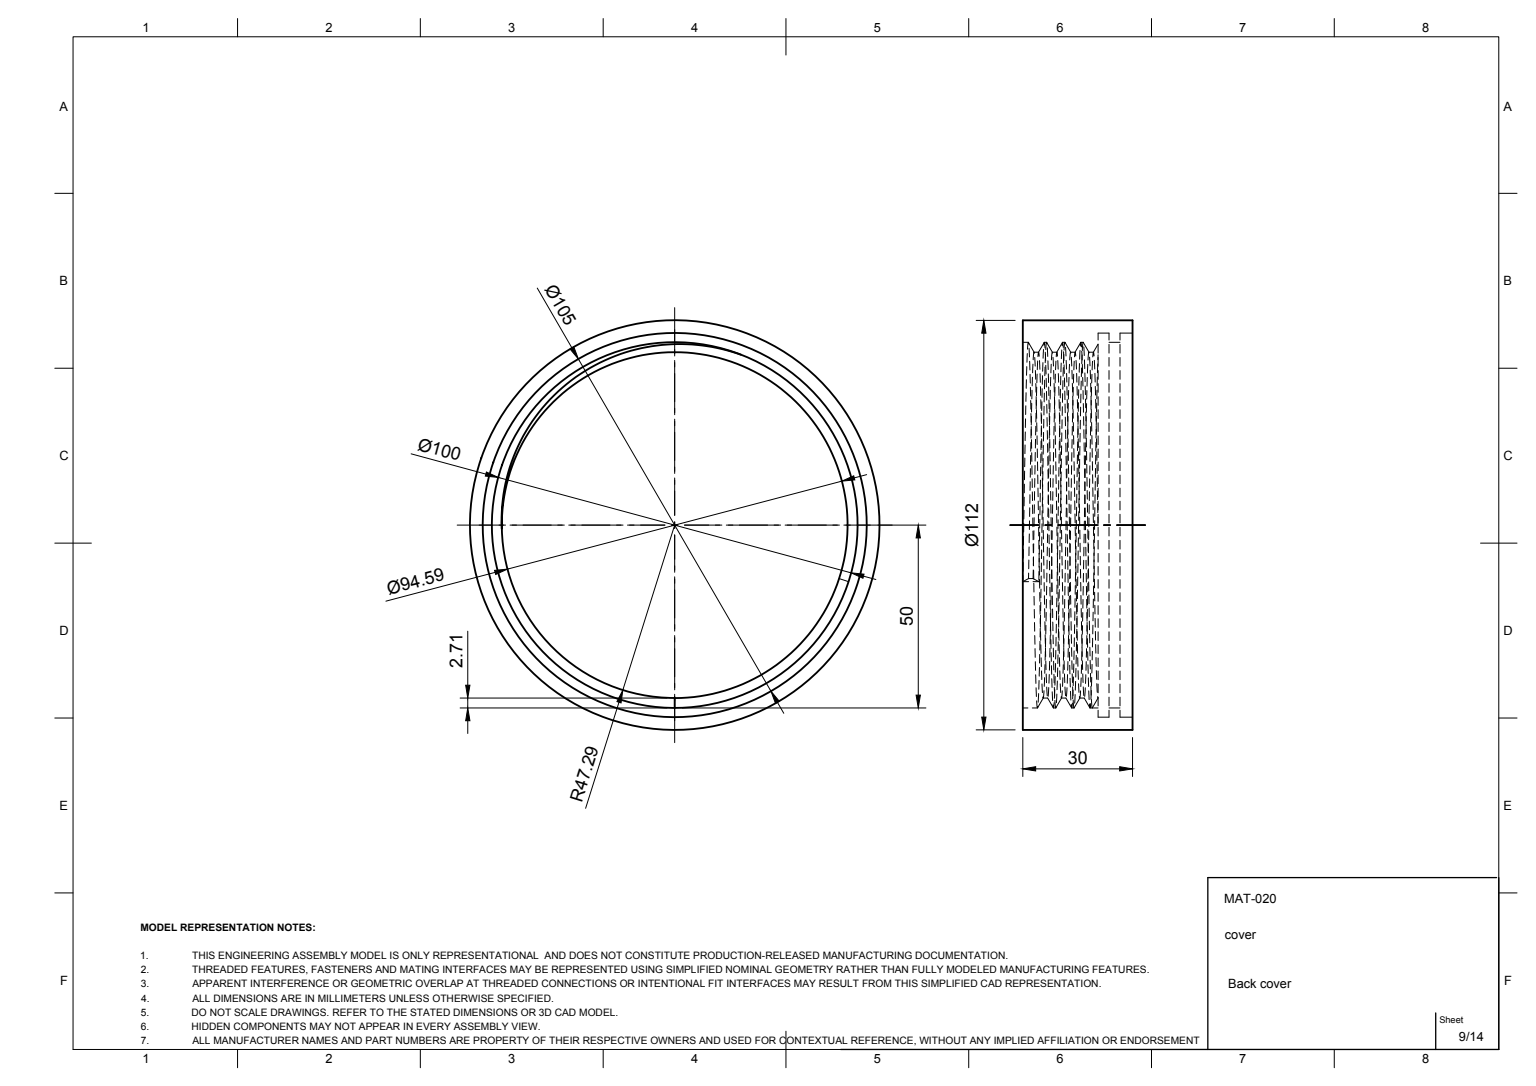
ISO-10303-21;
HEADER;
/* Generated by software containing ST-Developer
 * from STEP Tools, Inc. (www.steptools.com) 
 */

FILE_DESCRIPTION(
/* description */ ('STEP AP214'),
/* implementation_level */ '2;1');

FILE_NAME(
/* name */ 'Cover.step',
/* time_stamp */ '2026-11-14T06:20:50-08:00',
/* author */ (''),
/* organization */ (''),
/* preprocessor_version */ 'ST-DEVELOPER v20.2',
/* originating_system */ 'Autodesk Translation Framework v15.17.0.0',
/* authorisation */ '');

FILE_SCHEMA (('AUTOMOTIVE_DESIGN { 1 0 10303 214 3 1 1 }'));
ENDSEC;

DATA;
#10=MECHANICAL_DESIGN_GEOMETRIC_PRESENTATION_REPRESENTATION('',(#960),#20658);
#127=FACE_BOUND('',#1332,.T.);
#128=FACE_BOUND('',#1334,.T.);
#129=FACE_BOUND('',#1338,.T.);
#130=FACE_BOUND('',#1340,.T.);
#131=FACE_BOUND('',#1342,.T.);
#195=(
BOUNDED_SURFACE()
B_SPLINE_SURFACE(1,2,((#19897,#19898,#19899,#19900,#19901,#19902,#19903,
#19904,#19905,#19906,#19907,#19908,#19909,#19910,#19911,#19912,#19913,#19914,
#19915,#19916,#19917,#19918,#19919,#19920,#19921,#19922,#19923,#19924,#19925,
#19926,#19927,#19928,#19929,#19930,#19931,#19932,#19933,#19934,#19935,#19936,
#19937,#19938,#19939,#19940,#19941,#19942,#19943,#19944,#19945,#19946,#19947,
#19948,#19949,#19950,#19951,#19952,#19953,#19954,#19955,#19956,#19957,#19958,
#19959,#19960,#19961,#19962,#19963,#19964,#19965,#19966,#19967,#19968,#19969,
#19970,#19971,#19972,#19973,#19974,#19975,#19976,#19977,#19978,#19979,#19980,
#19981,#19982,#19983,#19984,#19985,#19986,#19987,#19988,#19989),(#19990,
#19991,#19992,#19993,#19994,#19995,#19996,#19997,#19998,#19999,#20000,#20001,
#20002,#20003,#20004,#20005,#20006,#20007,#20008,#20009,#20010,#20011,#20012,
#20013,#20014,#20015,#20016,#20017,#20018,#20019,#20020,#20021,#20022,#20023,
#20024,#20025,#20026,#20027,#20028,#20029,#20030,#20031,#20032,#20033,#20034,
#20035,#20036,#20037,#20038,#20039,#20040,#20041,#20042,#20043,#20044,#20045,
#20046,#20047,#20048,#20049,#20050,#20051,#20052,#20053,#20054,#20055,#20056,
#20057,#20058,#20059,#20060,#20061,#20062,#20063,#20064,#20065,#20066,#20067,
#20068,#20069,#20070,#20071,#20072,#20073,#20074,#20075,#20076,#20077,#20078,
#20079,#20080,#20081,#20082)),.UNSPECIFIED.,.F.,.F.,.F.)
B_SPLINE_SURFACE_WITH_KNOTS((2,2),(3,2,2,2,2,2,2,2,2,2,2,2,2,2,2,2,2,2,
2,2,2,2,2,2,2,2,2,2,2,2,2,2,2,2,2,2,2,2,2,2,2,2,2,2,2,2,3),(0.,1.),(0.,
0.0208333333333333,0.0416666666666667,0.0625,0.0833333333333333,0.104166666666667,
0.125,0.145833333333333,0.166666666666667,0.1875,0.208333333333333,0.229166666666667,
0.25,0.270833333333333,0.291666666666667,0.3125,0.333333333333333,0.354166666666667,
0.375,0.395833333333333,0.416666666666667,0.4375,0.458333333333333,0.479166666666667,
0.5,0.520833333333333,0.541666666666667,0.5625,0.583333333333333,0.604166666666667,
0.625,0.645833333333333,0.666666666666667,0.6875,0.708333333333333,0.729166666666667,
0.75,0.770833333333333,0.791666666666667,0.8125,0.833333333333333,0.854166666666667,
0.875,0.895833333333333,0.916666666666667,0.9375,0.949988556244299),
 .UNSPECIFIED.)
GEOMETRIC_REPRESENTATION_ITEM()
RATIONAL_B_SPLINE_SURFACE(((1.,0.965925826289068,1.,0.965925826289068,1.,
0.965925826289068,1.,0.965925826289068,1.,0.965925826289068,1.,0.965925826289068,
1.,0.965925826289068,1.,0.965925826289068,1.,0.965925826289068,1.,0.965925826289068,
1.,0.965925826289068,1.,0.965925826289068,1.,0.965925826289068,1.,0.965925826289068,
1.,0.965925826289068,1.,0.965925826289068,1.,0.965925826289068,1.,0.965925826289068,
1.,0.965925826289068,1.,0.965925826289068,1.,0.965925826289068,1.,0.965925826289068,
1.,0.965925826289068,1.,0.965925826289068,1.,0.965925826289068,1.,0.965925826289068,
1.,0.965925826289068,1.,0.965925826289068,1.,0.965925826289068,1.,0.965925826289068,
1.,0.965925826289068,1.,0.965925826289068,1.,0.965925826289068,1.,0.965925826289068,
1.,0.965925826289068,1.,0.965925826289068,1.,0.965925826289068,1.,0.965925826289068,
1.,0.965925826289068,1.,0.965925826289068,1.,0.965925826289068,1.,0.965925826289068,
1.,0.965925826289068,1.,0.965925826289068,1.,0.965925826289068,1.,0.979574212726385,
0.98363693040003),(1.,0.965925826289068,1.,0.965925826289068,1.,0.965925826289068,
1.,0.965925826289068,1.,0.965925826289068,1.,0.965925826289068,1.,0.965925826289068,
1.,0.965925826289068,1.,0.965925826289068,1.,0.965925826289068,1.,0.965925826289068,
1.,0.965925826289068,1.,0.965925826289068,1.,0.965925826289068,1.,0.965925826289068,
1.,0.965925826289068,1.,0.965925826289068,1.,0.965925826289068,1.,0.965925826289068,
1.,0.965925826289068,1.,0.965925826289068,1.,0.965925826289068,1.,0.965925826289068,
1.,0.965925826289068,1.,0.965925826289068,1.,0.965925826289068,1.,0.965925826289068,
1.,0.965925826289068,1.,0.965925826289068,1.,0.965925826289068,1.,0.965925826289068,
1.,0.965925826289068,1.,0.965925826289068,1.,0.965925826289068,1.,0.965925826289068,
1.,0.965925826289068,1.,0.965925826289068,1.,0.965925826289068,1.,0.965925826289068,
1.,0.965925826289068,1.,0.965925826289068,1.,0.965925826289068,1.,0.965925826289068,
1.,0.965925826289068,1.,0.965925826289068,1.,0.979574212726385,0.98363693040003)))
REPRESENTATION_ITEM('')
SURFACE()
);
#196=(
BOUNDED_SURFACE()
B_SPLINE_SURFACE(1,2,((#20106,#20107,#20108,#20109,#20110,#20111,#20112,
#20113,#20114,#20115,#20116,#20117,#20118,#20119,#20120,#20121,#20122,#20123,
#20124,#20125,#20126,#20127,#20128,#20129,#20130,#20131,#20132,#20133,#20134,
#20135,#20136,#20137,#20138,#20139,#20140,#20141,#20142,#20143,#20144,#20145,
#20146,#20147,#20148,#20149,#20150,#20151,#20152,#20153,#20154,#20155,#20156,
#20157,#20158,#20159,#20160,#20161,#20162,#20163,#20164,#20165,#20166,#20167,
#20168,#20169,#20170,#20171,#20172,#20173,#20174,#20175,#20176,#20177,#20178,
#20179,#20180,#20181,#20182,#20183,#20184,#20185,#20186,#20187,#20188,#20189,
#20190,#20191,#20192,#20193,#20194,#20195,#20196,#20197,#20198,#20199,#20200),
(#20201,#20202,#20203,#20204,#20205,#20206,#20207,#20208,#20209,#20210,
#20211,#20212,#20213,#20214,#20215,#20216,#20217,#20218,#20219,#20220,#20221,
#20222,#20223,#20224,#20225,#20226,#20227,#20228,#20229,#20230,#20231,#20232,
#20233,#20234,#20235,#20236,#20237,#20238,#20239,#20240,#20241,#20242,#20243,
#20244,#20245,#20246,#20247,#20248,#20249,#20250,#20251,#20252,#20253,#20254,
#20255,#20256,#20257,#20258,#20259,#20260,#20261,#20262,#20263,#20264,#20265,
#20266,#20267,#20268,#20269,#20270,#20271,#20272,#20273,#20274,#20275,#20276,
#20277,#20278,#20279,#20280,#20281,#20282,#20283,#20284,#20285,#20286,#20287,
#20288,#20289,#20290,#20291,#20292,#20293,#20294,#20295)),.UNSPECIFIED.,
 .F.,.F.,.F.)
B_SPLINE_SURFACE_WITH_KNOTS((2,2),(3,2,2,2,2,2,2,2,2,2,2,2,2,2,2,2,2,2,
2,2,2,2,2,2,2,2,2,2,2,2,2,2,2,2,2,2,2,2,2,2,2,2,2,2,2,2,2,3),(0.,1.),(0.,
0.0208333333333333,0.0416666666666667,0.0625,0.0833333333333333,0.104166666666667,
0.125,0.145833333333333,0.166666666666667,0.1875,0.208333333333333,0.229166666666667,
0.25,0.270833333333333,0.291666666666667,0.3125,0.333333333333333,0.354166666666667,
0.375,0.395833333333333,0.416666666666667,0.4375,0.458333333333333,0.479166666666667,
0.5,0.520833333333333,0.541666666666667,0.5625,0.583333333333333,0.604166666666667,
0.625,0.645833333333333,0.666666666666667,0.6875,0.708333333333333,0.729166666666667,
0.75,0.770833333333333,0.791666666666667,0.8125,0.833333333333333,0.854166666666667,
0.875,0.895833333333333,0.916666666666667,0.9375,0.949988555726961,0.95948844128423),
 .UNSPECIFIED.)
GEOMETRIC_REPRESENTATION_ITEM()
RATIONAL_B_SPLINE_SURFACE(((1.,0.965925826289068,1.,0.965925826289068,1.,
0.965925826289068,1.,0.965925826289068,1.,0.965925826289068,1.,0.965925826289068,
1.,0.965925826289068,1.,0.965925826289068,1.,0.965925826289068,1.,0.965925826289068,
1.,0.965925826289068,1.,0.965925826289068,1.,0.965925826289068,1.,0.965925826289068,
1.,0.965925826289068,1.,0.965925826289068,1.,0.965925826289068,1.,0.965925826289068,
1.,0.965925826289068,1.,0.965925826289068,1.,0.965925826289068,1.,0.965925826289068,
1.,0.965925826289068,1.,0.965925826289068,1.,0.965925826289068,1.,0.965925826289068,
1.,0.965925826289068,1.,0.965925826289068,1.,0.965925826289068,1.,0.965925826289068,
1.,0.965925826289068,1.,0.965925826289068,1.,0.965925826289068,1.,0.965925826289068,
1.,0.965925826289068,1.,0.965925826289068,1.,0.965925826289068,1.,0.965925826289068,
1.,0.965925826289068,1.,0.965925826289068,1.,0.965925826289068,1.,0.965925826289068,
1.,0.965925826289068,1.,0.965925826289068,1.,0.965925826289068,1.,0.979574213572523,
0.983636930063434,0.983636930063434,0.983636930063434),(1.,0.965925826289068,
1.,0.965925826289068,1.,0.965925826289068,1.,0.965925826289068,1.,0.965925826289068,
1.,0.965925826289068,1.,0.965925826289068,1.,0.965925826289068,1.,0.965925826289068,
1.,0.965925826289068,1.,0.965925826289068,1.,0.965925826289068,1.,0.965925826289068,
1.,0.965925826289068,1.,0.965925826289068,1.,0.965925826289068,1.,0.965925826289068,
1.,0.965925826289068,1.,0.965925826289068,1.,0.965925826289068,1.,0.965925826289068,
1.,0.965925826289068,1.,0.965925826289068,1.,0.965925826289068,1.,0.965925826289068,
1.,0.965925826289068,1.,0.965925826289068,1.,0.965925826289068,1.,0.965925826289068,
1.,0.965925826289068,1.,0.965925826289068,1.,0.965925826289068,1.,0.965925826289068,
1.,0.965925826289068,1.,0.965925826289068,1.,0.965925826289068,1.,0.965925826289068,
1.,0.965925826289068,1.,0.965925826289068,1.,0.965925826289068,1.,0.965925826289068,
1.,0.965925826289068,1.,0.965925826289068,1.,0.965925826289068,1.,0.965925826289068,
1.,0.979574213572523,0.983636930063434,0.983636930063434,0.983636930063434)))
REPRESENTATION_ITEM('')
SURFACE()
);
#282=(
BOUNDED_CURVE()
B_SPLINE_CURVE(2,(#19357,#19358,#19359),.UNSPECIFIED.,.F.,.F.)
B_SPLINE_CURVE_WITH_KNOTS((3,3),(0.921063726766605,0.935093935184017),
 .UNSPECIFIED.)
CURVE()
GEOMETRIC_REPRESENTATION_ITEM()
RATIONAL_B_SPLINE_CURVE((1.,0.978200372800764,0.98429423173899))
REPRESENTATION_ITEM('')
);
#283=(
BOUNDED_CURVE()
B_SPLINE_CURVE(2,(#19364,#19365,#19366,#19367,#19368,#19369,#19370,#19371,
#19372),.UNSPECIFIED.,.F.,.F.)
B_SPLINE_CURVE_WITH_KNOTS((3,2,2,2,3),(0.921063722504592,0.942993811135654,
0.964923899766715,0.986853988397777,0.999999994829099),.UNSPECIFIED.)
CURVE()
GEOMETRIC_REPRESENTATION_ITEM()
RATIONAL_B_SPLINE_CURVE((1.,0.965925826289068,1.,0.965925826289068,1.,0.965925826289068,
1.,0.979574221606877,0.98363692686735))
REPRESENTATION_ITEM('')
);
#284=(
BOUNDED_CURVE()
B_SPLINE_CURVE(2,(#19377,#19378,#19379,#19380,#19381,#19382,#19383,#19384,
#19385,#19386,#19387,#19388,#19389,#19390,#19391,#19392,#19393,#19394,#19395,
#19396,#19397,#19398,#19399,#19400,#19401),.UNSPECIFIED.,.F.,.F.)
B_SPLINE_CURVE_WITH_KNOTS((3,2,2,2,2,2,2,2,2,2,2,2,3),(0.657902661976146,
0.679832750708684,0.701762839441223,0.723692928173761,0.745623016906299,
0.767553105638837,0.789483194371375,0.811413283103914,0.833343371836452,
0.85527346056899,0.877203549301528,0.899133638034066,0.921063726766605),
 .UNSPECIFIED.)
CURVE()
GEOMETRIC_REPRESENTATION_ITEM()
RATIONAL_B_SPLINE_CURVE((1.,0.965925826289068,1.,0.965925826289068,1.,0.965925826289068,
1.,0.965925826289068,1.,0.965925826289068,1.,0.965925826289068,1.,0.965925826289068,
1.,0.965925826289068,1.,0.965925826289068,1.,0.965925826289068,1.,0.965925826289068,
1.,0.965925826289068,1.))
REPRESENTATION_ITEM('')
);
#285=(
BOUNDED_CURVE()
B_SPLINE_CURVE(2,(#19402,#19403,#19404,#19405,#19406,#19407,#19408,#19409,
#19410,#19411,#19412,#19413,#19414,#19415,#19416,#19417,#19418,#19419,#19420,
#19421,#19422,#19423,#19424,#19425,#19426),.UNSPECIFIED.,.F.,.F.)
B_SPLINE_CURVE_WITH_KNOTS((3,2,2,2,2,2,2,2,2,2,2,2,3),(0.657902658931851,
0.679832747562913,0.701762836193975,0.723692924825036,0.745623013456098,
0.76755310208716,0.789483190718221,0.811413279349283,0.833343367980345,
0.855273456611407,0.877203545242468,0.89913363387353,0.921063722504592),
 .UNSPECIFIED.)
CURVE()
GEOMETRIC_REPRESENTATION_ITEM()
RATIONAL_B_SPLINE_CURVE((1.,0.965925826289068,1.,0.965925826289068,1.,0.965925826289068,
1.,0.965925826289068,1.,0.965925826289068,1.,0.965925826289068,1.,0.965925826289068,
1.,0.965925826289068,1.,0.965925826289068,1.,0.965925826289068,1.,0.965925826289068,
1.,0.965925826289068,1.))
REPRESENTATION_ITEM('')
);
#286=(
BOUNDED_CURVE()
B_SPLINE_CURVE(2,(#19431,#19432,#19433,#19434,#19435,#19436,#19437,#19438,
#19439,#19440,#19441,#19442,#19443,#19444,#19445,#19446,#19447,#19448,#19449,
#19450,#19451,#19452,#19453,#19454,#19455),.UNSPECIFIED.,.F.,.F.)
B_SPLINE_CURVE_WITH_KNOTS((3,2,2,2,2,2,2,2,2,2,2,2,3),(0.394741597185688,
0.416671685918226,0.438601774650764,0.460531863383302,0.48246195211584,
0.504392040848379,0.526322129580917,0.548252218313455,0.570182307045993,
0.592112395778531,0.61404248451107,0.635972573243608,0.657902661976146),
 .UNSPECIFIED.)
CURVE()
GEOMETRIC_REPRESENTATION_ITEM()
RATIONAL_B_SPLINE_CURVE((1.,0.965925826289068,1.,0.965925826289068,1.,0.965925826289068,
1.,0.965925826289068,1.,0.965925826289068,1.,0.965925826289068,1.,0.965925826289068,
1.,0.965925826289068,1.,0.965925826289068,1.,0.965925826289068,1.,0.965925826289068,
1.,0.965925826289068,1.))
REPRESENTATION_ITEM('')
);
#287=(
BOUNDED_CURVE()
B_SPLINE_CURVE(2,(#19456,#19457,#19458,#19459,#19460,#19461,#19462,#19463,
#19464,#19465,#19466,#19467,#19468,#19469,#19470,#19471,#19472,#19473,#19474,
#19475,#19476,#19477,#19478,#19479,#19480),.UNSPECIFIED.,.F.,.F.)
B_SPLINE_CURVE_WITH_KNOTS((3,2,2,2,2,2,2,2,2,2,2,2,3),(0.394741595359111,
0.416671683990172,0.438601772621234,0.460531861252296,0.482461949883358,
0.504392038514419,0.526322127145481,0.548252215776543,0.570182304407604,
0.592112393038666,0.614042481669728,0.63597257030079,0.657902658931851),
 .UNSPECIFIED.)
CURVE()
GEOMETRIC_REPRESENTATION_ITEM()
RATIONAL_B_SPLINE_CURVE((1.,0.965925826289068,1.,0.965925826289068,1.,0.965925826289068,
1.,0.965925826289068,1.,0.965925826289068,1.,0.965925826289068,1.,0.965925826289068,
1.,0.965925826289068,1.,0.965925826289068,1.,0.965925826289068,1.,0.965925826289068,
1.,0.965925826289068,1.))
REPRESENTATION_ITEM('')
);
#288=(
BOUNDED_CURVE()
B_SPLINE_CURVE(2,(#19486,#19487,#19488,#19489,#19490,#19491,#19492,#19493,
#19494,#19495,#19496,#19497,#19498),.UNSPECIFIED.,.F.,.F.)
B_SPLINE_CURVE_WITH_KNOTS((3,2,2,2,2,2,3),(0.,0.0219300886310617,0.0438601772621234,
0.0657902658931851,0.0877203545242468,0.109650443155309,0.13158053178637),
 .UNSPECIFIED.)
CURVE()
GEOMETRIC_REPRESENTATION_ITEM()
RATIONAL_B_SPLINE_CURVE((1.,0.965925826289068,1.,0.965925826289068,1.,0.965925826289068,
1.,0.965925826289068,1.,0.965925826289068,1.,0.965925826289068,1.))
REPRESENTATION_ITEM('')
);
#289=(
BOUNDED_CURVE()
B_SPLINE_CURVE(2,(#19501,#19502,#19503,#19504,#19505,#19506,#19507,#19508,
#19509,#19510,#19511,#19512,#19513),.UNSPECIFIED.,.F.,.F.)
B_SPLINE_CURVE_WITH_KNOTS((3,2,2,2,2,2,3),(0.,0.0219300887325382,0.0438601774650764,
0.0657902661976146,0.0877203549301528,0.109650443662691,0.131580532395229),
 .UNSPECIFIED.)
CURVE()
GEOMETRIC_REPRESENTATION_ITEM()
RATIONAL_B_SPLINE_CURVE((1.,0.965925826289068,1.,0.965925826289068,1.,0.965925826289068,
1.,0.965925826289068,1.,0.965925826289068,1.,0.965925826289068,1.))
REPRESENTATION_ITEM('')
);
#290=(
BOUNDED_CURVE()
B_SPLINE_CURVE(2,(#19847,#19848,#19849,#19850,#19851,#19852,#19853,#19854,
#19855,#19856,#19857,#19858,#19859,#19860,#19861,#19862,#19863,#19864,#19865,
#19866,#19867,#19868,#19869,#19870,#19871),.UNSPECIFIED.,.F.,.F.)
B_SPLINE_CURVE_WITH_KNOTS((3,2,2,2,2,2,2,2,2,2,2,2,3),(0.131580532395229,
0.153510621127767,0.175440709860306,0.197370798592844,0.219300887325382,
0.24123097605792,0.263161064790458,0.285091153522997,0.307021242255535,
0.328951330988073,0.350881419720611,0.372811508453149,0.394741597185688),
 .UNSPECIFIED.)
CURVE()
GEOMETRIC_REPRESENTATION_ITEM()
RATIONAL_B_SPLINE_CURVE((1.,0.965925826289068,1.,0.965925826289068,1.,0.965925826289068,
1.,0.965925826289068,1.,0.965925826289068,1.,0.965925826289068,1.,0.965925826289068,
1.,0.965925826289068,1.,0.965925826289068,1.,0.965925826289068,1.,0.965925826289068,
1.,0.965925826289068,1.))
REPRESENTATION_ITEM('')
);
#291=(
BOUNDED_CURVE()
B_SPLINE_CURVE(2,(#19872,#19873,#19874,#19875,#19876,#19877,#19878,#19879,
#19880,#19881,#19882,#19883,#19884,#19885,#19886,#19887,#19888,#19889,#19890,
#19891,#19892,#19893,#19894,#19895,#19896),.UNSPECIFIED.,.F.,.F.)
B_SPLINE_CURVE_WITH_KNOTS((3,2,2,2,2,2,2,2,2,2,2,2,3),(0.13158053178637,
0.153510620417432,0.175440709048494,0.197370797679555,0.219300886310617,
0.241230974941679,0.26316106357274,0.285091152203802,0.307021240834864,
0.328951329465926,0.350881418096987,0.372811506728049,0.394741595359111),
 .UNSPECIFIED.)
CURVE()
GEOMETRIC_REPRESENTATION_ITEM()
RATIONAL_B_SPLINE_CURVE((1.,0.965925826289068,1.,0.965925826289068,1.,0.965925826289068,
1.,0.965925826289068,1.,0.965925826289068,1.,0.965925826289068,1.,0.965925826289068,
1.,0.965925826289068,1.,0.965925826289068,1.,0.965925826289068,1.,0.965925826289068,
1.,0.965925826289068,1.))
REPRESENTATION_ITEM('')
);
#381=B_SPLINE_CURVE_WITH_KNOTS('',3,(#19520,#19521,#19522,#19523,#19524,
#19525,#19526,#19527,#19528,#19529,#19530,#19531,#19532,#19533,#19534,#19535,
#19536,#19537,#19538,#19539,#19540,#19541,#19542,#19543,#19544,#19545,#19546,
#19547),.UNSPECIFIED.,.F.,.F.,(4,2,2,2,2,2,2,2,2,2,2,2,2,4),(0.,1.30396391294989,
2.60816609231495,4.56086018974018,6.500232979704,8.45070313715037,10.4269067443957,
12.3773244878899,14.3166724219264,16.2692988357265,18.2429971279301,20.1912804500865,
22.1308341479624,23.6343466236277),.UNSPECIFIED.);
#382=B_SPLINE_CURVE_WITH_KNOTS('',3,(#19553,#19554,#19555,#19556,#19557,
#19558,#19559,#19560,#19561,#19562,#19563,#19564,#19565,#19566,#19567,#19568,
#19569,#19570,#19571,#19572,#19573,#19574,#19575,#19576,#19577,#19578,#19579,
#19580),.UNSPECIFIED.,.F.,.F.,(4,2,2,2,2,2,2,2,2,2,2,2,2,4),(78.502201789525,
80.3928667388685,82.3384972109937,84.2788241322494,86.2377173630452,88.2079834738884,
90.1520350835772,92.0931180658711,94.0544724803042,96.0212222485092,97.9638912741162,
99.9059931283975,101.023430324553,102.135964763307),.UNSPECIFIED.);
#383=B_SPLINE_CURVE_WITH_KNOTS('',3,(#19583,#19584,#19585,#19586,#19587,
#19588,#19589,#19590,#19591,#19592,#19593,#19594,#19595,#19596,#19597,#19598,
#19599,#19600,#19601,#19602,#19603,#19604,#19605,#19606,#19607,#19608,#19609,
#19610,#19611,#19612,#19613,#19614,#19615,#19616,#19617,#19618),
 .UNSPECIFIED.,.F.,.F.,(4,2,2,2,2,2,2,2,2,2,2,2,2,2,2,2,2,4),(23.6343466236277,
24.0859013362698,26.0570400286112,28.003370843106,29.9433774048251,31.9011613014351,
33.869710627465,35.8143050082161,37.7550192764481,39.7157770489108,41.6817334338505,
43.6248336037104,45.5665083217582,47.5304684261993,49.4938551346482,51.435719911611,
53.3785958965145,55.1510718902642),.UNSPECIFIED.);
#384=B_SPLINE_CURVE_WITH_KNOTS('',3,(#19623,#19624,#19625,#19626,#19627,
#19628,#19629,#19630,#19631,#19632,#19633,#19634,#19635,#19636,#19637,#19638,
#19639,#19640,#19641,#19642,#19643,#19644,#19645,#19646,#19647,#19648,#19649,
#19650,#19651,#19652,#19653,#19654,#19655,#19656,#19657,#19658,#19659,#19660),
 .UNSPECIFIED.,.F.,.F.,(4,2,2,2,2,2,2,2,2,2,2,2,2,2,2,2,2,2,4),(46.9842134144311,
47.1683179476468,49.128813348479,51.0696211747879,53.0090557646061,54.9587871273889,
56.9342063154586,58.8854100779273,60.8247947630869,62.7767598037459,64.7546358588809,
66.7038727383019,68.6434231351511,70.5976920946369,72.575259116529,74.5226306638379,
76.4624530680027,78.418977906567,78.502201789525),.UNSPECIFIED.);
#385=B_SPLINE_CURVE_WITH_KNOTS('',3,(#19661,#19662,#19663,#19664,#19665,
#19666,#19667,#19668,#19669,#19670,#19671,#19672,#19673,#19674,#19675,#19676,
#19677,#19678,#19679,#19680,#19681,#19682,#19683,#19684,#19685,#19686,#19687,
#19688,#19689,#19690,#19691,#19692,#19693,#19694,#19695,#19696,#19697,#19698),
 .UNSPECIFIED.,.F.,.F.,(4,2,2,2,2,2,2,2,2,2,2,2,2,2,2,2,2,2,4),(55.1510718902642,
55.3459492191646,57.3068158150841,59.2477103486072,61.1871252191665,63.1364287476564,
65.1113578818397,67.0628817695785,69.0022066891439,70.953719601354,72.9311191528217,
74.8806267146135,76.8200815012103,78.7738929823442,80.7520431717114,82.6996675386312,
84.6393555394773,86.5954010716407,86.6680978070119),.UNSPECIFIED.);
#386=B_SPLINE_CURVE_WITH_KNOTS('',3,(#19704,#19705,#19706,#19707,#19708,
#19709,#19710,#19711,#19712,#19713,#19714,#19715,#19716,#19717,#19718,#19719,
#19720,#19721),.UNSPECIFIED.,.F.,.F.,(4,2,2,2,2,2,2,2,4),(118.184020883807,
118.803694236851,119.279145252132,119.517336391626,119.636434572161,119.695970056689,
119.725732617238,119.740612379807,119.756924319264),.UNSPECIFIED.);
#387=B_SPLINE_CURVE_WITH_KNOTS('',3,(#19726,#19727,#19728,#19729,#19730,
#19731,#19732,#19733,#19734,#19735,#19736,#19737,#19738,#19739,#19740,#19741,
#19742,#19743,#19744,#19745),.UNSPECIFIED.,.F.,.F.,(4,2,2,2,2,2,2,2,2,4),
(9.99999992304919E-7,1.12538984857621,2.24819806101112,4.19829220265297,
6.13771124438825,8.09078865884484,10.0641056167008,12.0120937201665,13.9517598952885,
15.4666452689729),.UNSPECIFIED.);
#388=B_SPLINE_CURVE_WITH_KNOTS('',3,(#19771,#19772,#19773,#19774,#19775,
#19776,#19777,#19778,#19779,#19780,#19781,#19782,#19783,#19784,#19785,#19786,
#19787,#19788,#19789,#19790,#19791,#19792,#19793,#19794,#19795,#19796,#19797,
#19798,#19799,#19800,#19801,#19802,#19803,#19804,#19805,#19806),
 .UNSPECIFIED.,.F.,.F.,(4,2,2,2,2,2,2,2,2,2,2,2,2,2,2,2,2,4),(15.4666452689729,
15.9073263138292,17.8780768344747,19.8241472733818,21.7643097977368,23.7226387447498,
25.690797326506,27.6351711527205,29.576085113709,31.5374294358844,33.5029970868268,
35.4459200800723,37.3878368573986,39.35241917033,41.3154237226985,43.2571565265499,
45.2003139491873,46.9842134144311),.UNSPECIFIED.);
#389=B_SPLINE_CURVE_WITH_KNOTS('',3,(#19807,#19808,#19809,#19810,#19811,
#19812,#19813,#19814,#19815,#19816,#19817,#19818,#19819,#19820,#19821,#19822,
#19823,#19824,#19825,#19826,#19827,#19828,#19829,#19830,#19831,#19832,#19833,
#19834,#19835,#19836,#19837,#19838,#19839,#19840,#19841,#19842),
 .UNSPECIFIED.,.F.,.F.,(4,2,2,2,2,2,2,2,2,2,2,2,2,2,2,2,2,4),(86.6680978070119,
88.5698686964051,90.5157271678372,92.4558768432157,94.4142720649564,96.3851035202131,
98.329351784228,100.27021180681,102.231053249456,104.198345974643,106.141174650795,
108.083006466375,110.046368338904,112.010268920263,113.951897726735,115.894966472163,
117.860898185085,118.184020883807),.UNSPECIFIED.);
#390=B_SPLINE_CURVE_WITH_KNOTS('',3,(#20083,#20084,#20085,#20086,#20087,
#20088,#20089,#20090,#20091,#20092,#20093,#20094,#20095,#20096,#20097,#20098,
#20099,#20100),.UNSPECIFIED.,.F.,.F.,(4,2,2,2,2,2,2,2,4),(0.,0.978481252991969,
1.98438926043037,3.83556386007751,4.8022813892872,5.7579599217032,7.83058544513618,
8.89308643237631,9.98441482005272),.UNSPECIFIED.);
#415=PLANE('',#3958);
#416=PLANE('',#3960);
#417=PLANE('',#3961);
#418=PLANE('',#3962);
#419=PLANE('',#3963);
#420=PLANE('',#3964);
#421=PLANE('',#3965);
#572=LINE('',#19355,#765);
#573=LINE('',#19363,#766);
#574=LINE('',#19376,#767);
#575=LINE('',#19430,#768);
#576=LINE('',#19484,#769);
#577=LINE('',#19500,#770);
#578=LINE('',#19517,#771);
#579=LINE('',#19551,#772);
#580=LINE('',#19581,#773);
#581=LINE('',#19622,#774);
#582=LINE('',#19702,#775);
#583=LINE('',#19723,#776);
#584=LINE('',#19750,#777);
#585=LINE('',#19756,#778);
#586=LINE('',#19762,#779);
#587=LINE('',#19768,#780);
#588=LINE('',#19844,#781);
#589=LINE('',#19845,#782);
#590=LINE('',#20101,#783);
#591=LINE('',#20105,#784);
#765=VECTOR('',#4529,47.293670625);
#766=VECTOR('',#4532,10.);
#767=VECTOR('',#4535,47.293670625);
#768=VECTOR('',#4538,47.293670625);
#769=VECTOR('',#4541,47.293670625);
#770=VECTOR('',#4542,10.);
#771=VECTOR('',#4545,50.);
#772=VECTOR('',#4550,50.);
#773=VECTOR('',#4551,1000.);
#774=VECTOR('',#4556,50.);
#775=VECTOR('',#4559,50.);
#776=VECTOR('',#4560,1000.);
#777=VECTOR('',#4567,52.5);
#778=VECTOR('',#4574,52.5);
#779=VECTOR('',#4581,56.);
#780=VECTOR('',#4588,50.);
#781=VECTOR('',#4595,1000.);
#782=VECTOR('',#4596,10.);
#783=VECTOR('',#4599,10.);
#784=VECTOR('',#4606,10.);
#891=CYLINDRICAL_SURFACE('',#3933,47.293670625);
#892=CYLINDRICAL_SURFACE('',#3935,47.293670625);
#893=CYLINDRICAL_SURFACE('',#3936,47.293670625);
#894=CYLINDRICAL_SURFACE('',#3937,47.293670625);
#895=CYLINDRICAL_SURFACE('',#3938,50.);
#896=CYLINDRICAL_SURFACE('',#3940,50.);
#897=CYLINDRICAL_SURFACE('',#3942,50.);
#898=CYLINDRICAL_SURFACE('',#3943,50.);
#899=CYLINDRICAL_SURFACE('',#3945,52.5);
#900=CYLINDRICAL_SURFACE('',#3948,52.5);
#901=CYLINDRICAL_SURFACE('',#3951,56.);
#902=CYLINDRICAL_SURFACE('',#3954,50.);
#903=CYLINDRICAL_SURFACE('',#3957,50.);
#904=CYLINDRICAL_SURFACE('',#3959,47.293670625);
#936=SHAPE_REPRESENTATION_RELATIONSHIP('SRR','None',#20720,#948);
#948=ADVANCED_BREP_SHAPE_REPRESENTATION('',(#972),#20650);
#960=STYLED_ITEM('',(#20787),#972);
#972=MANIFOLD_SOLID_BREP('Body1',#3655);
#1103=FACE_OUTER_BOUND('',#1315,.T.);
#1104=FACE_OUTER_BOUND('',#1316,.T.);
#1105=FACE_OUTER_BOUND('',#1317,.T.);
#1106=FACE_OUTER_BOUND('',#1318,.T.);
#1107=FACE_OUTER_BOUND('',#1319,.T.);
#1108=FACE_OUTER_BOUND('',#1320,.T.);
#1109=FACE_OUTER_BOUND('',#1321,.T.);
#1110=FACE_OUTER_BOUND('',#1322,.T.);
#1111=FACE_OUTER_BOUND('',#1323,.T.);
#1112=FACE_OUTER_BOUND('',#1324,.T.);
#1113=FACE_OUTER_BOUND('',#1325,.T.);
#1114=FACE_OUTER_BOUND('',#1326,.T.);
#1115=FACE_OUTER_BOUND('',#1327,.T.);
#1116=FACE_OUTER_BOUND('',#1328,.T.);
#1117=FACE_OUTER_BOUND('',#1329,.T.);
#1118=FACE_OUTER_BOUND('',#1330,.T.);
#1119=FACE_OUTER_BOUND('',#1331,.T.);
#1120=FACE_OUTER_BOUND('',#1333,.T.);
#1121=FACE_OUTER_BOUND('',#1335,.T.);
#1122=FACE_OUTER_BOUND('',#1336,.T.);
#1123=FACE_OUTER_BOUND('',#1337,.T.);
#1124=FACE_OUTER_BOUND('',#1339,.T.);
#1125=FACE_OUTER_BOUND('',#1341,.T.);
#1315=EDGE_LOOP('',(#3096,#3097,#3098,#3099,#3100));
#1316=EDGE_LOOP('',(#3101,#3102,#3103,#3104));
#1317=EDGE_LOOP('',(#3105,#3106,#3107,#3108));
#1318=EDGE_LOOP('',(#3109,#3110,#3111,#3112));
#1319=EDGE_LOOP('',(#3113,#3114,#3115));
#1320=EDGE_LOOP('',(#3116,#3117,#3118,#3119,#3120,#3121));
#1321=EDGE_LOOP('',(#3122,#3123,#3124,#3125));
#1322=EDGE_LOOP('',(#3126,#3127,#3128,#3129,#3130));
#1323=EDGE_LOOP('',(#3131,#3132,#3133,#3134));
#1324=EDGE_LOOP('',(#3135,#3136,#3137,#3138));
#1325=EDGE_LOOP('',(#3139,#3140,#3141,#3142));
#1326=EDGE_LOOP('',(#3143,#3144,#3145,#3146));
#1327=EDGE_LOOP('',(#3147,#3148,#3149,#3150));
#1328=EDGE_LOOP('',(#3151,#3152,#3153,#3154));
#1329=EDGE_LOOP('',(#3155,#3156,#3157,#3158));
#1330=EDGE_LOOP('',(#3159,#3160,#3161,#3162,#3163,#3164,#3165,#3166,#3167,
#3168,#3169));
#1331=EDGE_LOOP('',(#3170));
#1332=EDGE_LOOP('',(#3171));
#1333=EDGE_LOOP('',(#3172));
#1334=EDGE_LOOP('',(#3173,#3174));
#1335=EDGE_LOOP('',(#3175,#3176,#3177,#3178));
#1336=EDGE_LOOP('',(#3179,#3180,#3181,#3182,#3183,#3184,#3185,#3186,#3187,
#3188,#3189,#3190));
#1337=EDGE_LOOP('',(#3191));
#1338=EDGE_LOOP('',(#3192));
#1339=EDGE_LOOP('',(#3193));
#1340=EDGE_LOOP('',(#3194,#3195,#3196,#3197));
#1341=EDGE_LOOP('',(#3198));
#1342=EDGE_LOOP('',(#3199));
#1471=CIRCLE('',#3934,47.293670625);
#1472=CIRCLE('',#3939,50.);
#1473=CIRCLE('',#3941,50.);
#1474=CIRCLE('',#3944,50.);
#1475=CIRCLE('',#3946,52.5);
#1476=CIRCLE('',#3947,52.5);
#1477=CIRCLE('',#3949,52.5);
#1478=CIRCLE('',#3950,52.5);
#1479=CIRCLE('',#3952,56.);
#1480=CIRCLE('',#3953,56.);
#1481=CIRCLE('',#3955,50.);
#1482=CIRCLE('',#3956,50.);
#1777=VERTEX_POINT('',#19353);
#1778=VERTEX_POINT('',#19354);
#1779=VERTEX_POINT('',#19356);
#1780=VERTEX_POINT('',#19360);
#1781=VERTEX_POINT('',#19362);
#1782=VERTEX_POINT('',#19374);
#1783=VERTEX_POINT('',#19375);
#1784=VERTEX_POINT('',#19428);
#1785=VERTEX_POINT('',#19429);
#1786=VERTEX_POINT('',#19482);
#1787=VERTEX_POINT('',#19483);
#1788=VERTEX_POINT('',#19485);
#1789=VERTEX_POINT('',#19499);
#1790=VERTEX_POINT('',#19515);
#1791=VERTEX_POINT('',#19516);
#1792=VERTEX_POINT('',#19518);
#1793=VERTEX_POINT('',#19549);
#1794=VERTEX_POINT('',#19550);
#1795=VERTEX_POINT('',#19552);
#1796=VERTEX_POINT('',#19620);
#1797=VERTEX_POINT('',#19621);
#1798=VERTEX_POINT('',#19700);
#1799=VERTEX_POINT('',#19701);
#1800=VERTEX_POINT('',#19703);
#1801=VERTEX_POINT('',#19722);
#1802=VERTEX_POINT('',#19724);
#1803=VERTEX_POINT('',#19747);
#1804=VERTEX_POINT('',#19749);
#1805=VERTEX_POINT('',#19753);
#1806=VERTEX_POINT('',#19755);
#1807=VERTEX_POINT('',#19759);
#1808=VERTEX_POINT('',#19761);
#1809=VERTEX_POINT('',#19765);
#1810=VERTEX_POINT('',#19767);
#2230=EDGE_CURVE('',#1777,#1778,#572,.T.);
#2231=EDGE_CURVE('',#1778,#1779,#282,.T.);
#2232=EDGE_CURVE('',#1780,#1779,#1471,.T.);
#2233=EDGE_CURVE('',#1781,#1780,#573,.T.);
#2234=EDGE_CURVE('',#1777,#1781,#283,.T.);
#2235=EDGE_CURVE('',#1782,#1783,#574,.T.);
#2236=EDGE_CURVE('',#1783,#1778,#284,.T.);
#2237=EDGE_CURVE('',#1782,#1777,#285,.T.);
#2238=EDGE_CURVE('',#1784,#1785,#575,.T.);
#2239=EDGE_CURVE('',#1785,#1783,#286,.T.);
#2240=EDGE_CURVE('',#1784,#1782,#287,.T.);
#2241=EDGE_CURVE('',#1786,#1787,#576,.T.);
#2242=EDGE_CURVE('',#1788,#1786,#288,.T.);
#2243=EDGE_CURVE('',#1789,#1788,#577,.T.);
#2244=EDGE_CURVE('',#1789,#1787,#289,.T.);
#2245=EDGE_CURVE('',#1790,#1791,#578,.T.);
#2246=EDGE_CURVE('',#1792,#1791,#1472,.T.);
#2247=EDGE_CURVE('',#1792,#1790,#381,.T.);
#2248=EDGE_CURVE('',#1793,#1794,#579,.T.);
#2249=EDGE_CURVE('',#1795,#1794,#382,.F.);
#2250=EDGE_CURVE('',#1792,#1795,#580,.T.);
#2251=EDGE_CURVE('',#1791,#1792,#1473,.T.);
#2252=EDGE_CURVE('',#1790,#1793,#383,.T.);
#2253=EDGE_CURVE('',#1796,#1797,#581,.T.);
#2254=EDGE_CURVE('',#1794,#1797,#384,.F.);
#2255=EDGE_CURVE('',#1793,#1796,#385,.T.);
#2256=EDGE_CURVE('',#1798,#1799,#582,.T.);
#2257=EDGE_CURVE('',#1798,#1800,#386,.T.);
#2258=EDGE_CURVE('',#1801,#1800,#583,.T.);
#2259=EDGE_CURVE('',#1801,#1802,#1474,.T.);
#2260=EDGE_CURVE('',#1799,#1802,#387,.F.);
#2261=EDGE_CURVE('',#1803,#1803,#1475,.T.);
#2262=EDGE_CURVE('',#1803,#1804,#584,.T.);
#2263=EDGE_CURVE('',#1804,#1804,#1476,.T.);
#2264=EDGE_CURVE('',#1805,#1805,#1477,.T.);
#2265=EDGE_CURVE('',#1805,#1806,#585,.T.);
#2266=EDGE_CURVE('',#1806,#1806,#1478,.T.);
#2267=EDGE_CURVE('',#1807,#1807,#1479,.T.);
#2268=EDGE_CURVE('',#1807,#1808,#586,.T.);
#2269=EDGE_CURVE('',#1808,#1808,#1480,.T.);
#2270=EDGE_CURVE('',#1809,#1809,#1481,.T.);
#2271=EDGE_CURVE('',#1809,#1810,#587,.T.);
#2272=EDGE_CURVE('',#1810,#1810,#1482,.T.);
#2273=EDGE_CURVE('',#1797,#1799,#388,.F.);
#2274=EDGE_CURVE('',#1796,#1798,#389,.T.);
#2275=EDGE_CURVE('',#1801,#1780,#588,.T.);
#2276=EDGE_CURVE('',#1800,#1781,#589,.T.);
#2277=EDGE_CURVE('',#1787,#1785,#290,.T.);
#2278=EDGE_CURVE('',#1786,#1784,#291,.T.);
#2279=EDGE_CURVE('',#1779,#1802,#390,.T.);
#2280=EDGE_CURVE('',#1795,#1789,#590,.T.);
#2281=EDGE_CURVE('',#1788,#1792,#591,.T.);
#3096=ORIENTED_EDGE('',*,*,#2230,.T.);
#3097=ORIENTED_EDGE('',*,*,#2231,.T.);
#3098=ORIENTED_EDGE('',*,*,#2232,.F.);
#3099=ORIENTED_EDGE('',*,*,#2233,.F.);
#3100=ORIENTED_EDGE('',*,*,#2234,.F.);
#3101=ORIENTED_EDGE('',*,*,#2235,.T.);
#3102=ORIENTED_EDGE('',*,*,#2236,.T.);
#3103=ORIENTED_EDGE('',*,*,#2230,.F.);
#3104=ORIENTED_EDGE('',*,*,#2237,.F.);
#3105=ORIENTED_EDGE('',*,*,#2238,.T.);
#3106=ORIENTED_EDGE('',*,*,#2239,.T.);
#3107=ORIENTED_EDGE('',*,*,#2235,.F.);
#3108=ORIENTED_EDGE('',*,*,#2240,.F.);
#3109=ORIENTED_EDGE('',*,*,#2241,.F.);
#3110=ORIENTED_EDGE('',*,*,#2242,.F.);
#3111=ORIENTED_EDGE('',*,*,#2243,.F.);
#3112=ORIENTED_EDGE('',*,*,#2244,.T.);
#3113=ORIENTED_EDGE('',*,*,#2245,.T.);
#3114=ORIENTED_EDGE('',*,*,#2246,.F.);
#3115=ORIENTED_EDGE('',*,*,#2247,.T.);
#3116=ORIENTED_EDGE('',*,*,#2248,.T.);
#3117=ORIENTED_EDGE('',*,*,#2249,.F.);
#3118=ORIENTED_EDGE('',*,*,#2250,.F.);
#3119=ORIENTED_EDGE('',*,*,#2251,.F.);
#3120=ORIENTED_EDGE('',*,*,#2245,.F.);
#3121=ORIENTED_EDGE('',*,*,#2252,.T.);
#3122=ORIENTED_EDGE('',*,*,#2253,.T.);
#3123=ORIENTED_EDGE('',*,*,#2254,.F.);
#3124=ORIENTED_EDGE('',*,*,#2248,.F.);
#3125=ORIENTED_EDGE('',*,*,#2255,.T.);
#3126=ORIENTED_EDGE('',*,*,#2256,.F.);
#3127=ORIENTED_EDGE('',*,*,#2257,.T.);
#3128=ORIENTED_EDGE('',*,*,#2258,.F.);
#3129=ORIENTED_EDGE('',*,*,#2259,.T.);
#3130=ORIENTED_EDGE('',*,*,#2260,.F.);
#3131=ORIENTED_EDGE('',*,*,#2261,.F.);
#3132=ORIENTED_EDGE('',*,*,#2262,.T.);
#3133=ORIENTED_EDGE('',*,*,#2263,.T.);
#3134=ORIENTED_EDGE('',*,*,#2262,.F.);
#3135=ORIENTED_EDGE('',*,*,#2264,.F.);
#3136=ORIENTED_EDGE('',*,*,#2265,.T.);
#3137=ORIENTED_EDGE('',*,*,#2266,.T.);
#3138=ORIENTED_EDGE('',*,*,#2265,.F.);
#3139=ORIENTED_EDGE('',*,*,#2267,.T.);
#3140=ORIENTED_EDGE('',*,*,#2268,.T.);
#3141=ORIENTED_EDGE('',*,*,#2269,.F.);
#3142=ORIENTED_EDGE('',*,*,#2268,.F.);
#3143=ORIENTED_EDGE('',*,*,#2270,.T.);
#3144=ORIENTED_EDGE('',*,*,#2271,.T.);
#3145=ORIENTED_EDGE('',*,*,#2272,.F.);
#3146=ORIENTED_EDGE('',*,*,#2271,.F.);
#3147=ORIENTED_EDGE('',*,*,#2256,.T.);
#3148=ORIENTED_EDGE('',*,*,#2273,.F.);
#3149=ORIENTED_EDGE('',*,*,#2253,.F.);
#3150=ORIENTED_EDGE('',*,*,#2274,.T.);
#3151=ORIENTED_EDGE('',*,*,#2275,.F.);
#3152=ORIENTED_EDGE('',*,*,#2258,.T.);
#3153=ORIENTED_EDGE('',*,*,#2276,.T.);
#3154=ORIENTED_EDGE('',*,*,#2233,.T.);
#3155=ORIENTED_EDGE('',*,*,#2241,.T.);
#3156=ORIENTED_EDGE('',*,*,#2277,.T.);
#3157=ORIENTED_EDGE('',*,*,#2238,.F.);
#3158=ORIENTED_EDGE('',*,*,#2278,.F.);
#3159=ORIENTED_EDGE('',*,*,#2279,.F.);
#3160=ORIENTED_EDGE('',*,*,#2231,.F.);
#3161=ORIENTED_EDGE('',*,*,#2236,.F.);
#3162=ORIENTED_EDGE('',*,*,#2239,.F.);
#3163=ORIENTED_EDGE('',*,*,#2277,.F.);
#3164=ORIENTED_EDGE('',*,*,#2244,.F.);
#3165=ORIENTED_EDGE('',*,*,#2280,.F.);
#3166=ORIENTED_EDGE('',*,*,#2249,.T.);
#3167=ORIENTED_EDGE('',*,*,#2254,.T.);
#3168=ORIENTED_EDGE('',*,*,#2273,.T.);
#3169=ORIENTED_EDGE('',*,*,#2260,.T.);
#3170=ORIENTED_EDGE('',*,*,#2269,.T.);
#3171=ORIENTED_EDGE('',*,*,#2266,.F.);
#3172=ORIENTED_EDGE('',*,*,#2267,.F.);
#3173=ORIENTED_EDGE('',*,*,#2246,.T.);
#3174=ORIENTED_EDGE('',*,*,#2251,.T.);
#3175=ORIENTED_EDGE('',*,*,#2281,.T.);
#3176=ORIENTED_EDGE('',*,*,#2250,.T.);
#3177=ORIENTED_EDGE('',*,*,#2280,.T.);
#3178=ORIENTED_EDGE('',*,*,#2243,.T.);
#3179=ORIENTED_EDGE('',*,*,#2281,.F.);
#3180=ORIENTED_EDGE('',*,*,#2242,.T.);
#3181=ORIENTED_EDGE('',*,*,#2278,.T.);
#3182=ORIENTED_EDGE('',*,*,#2240,.T.);
#3183=ORIENTED_EDGE('',*,*,#2237,.T.);
#3184=ORIENTED_EDGE('',*,*,#2234,.T.);
#3185=ORIENTED_EDGE('',*,*,#2276,.F.);
#3186=ORIENTED_EDGE('',*,*,#2257,.F.);
#3187=ORIENTED_EDGE('',*,*,#2274,.F.);
#3188=ORIENTED_EDGE('',*,*,#2255,.F.);
#3189=ORIENTED_EDGE('',*,*,#2252,.F.);
#3190=ORIENTED_EDGE('',*,*,#2247,.F.);
#3191=ORIENTED_EDGE('',*,*,#2264,.T.);
#3192=ORIENTED_EDGE('',*,*,#2270,.F.);
#3193=ORIENTED_EDGE('',*,*,#2261,.T.);
#3194=ORIENTED_EDGE('',*,*,#2275,.T.);
#3195=ORIENTED_EDGE('',*,*,#2232,.T.);
#3196=ORIENTED_EDGE('',*,*,#2279,.T.);
#3197=ORIENTED_EDGE('',*,*,#2259,.F.);
#3198=ORIENTED_EDGE('',*,*,#2263,.F.);
#3199=ORIENTED_EDGE('',*,*,#2272,.T.);
#3565=ADVANCED_FACE('',(#1103),#891,.F.);
#3566=ADVANCED_FACE('',(#1104),#892,.F.);
#3567=ADVANCED_FACE('',(#1105),#893,.F.);
#3568=ADVANCED_FACE('',(#1106),#894,.F.);
#3569=ADVANCED_FACE('',(#1107),#895,.F.);
#3570=ADVANCED_FACE('',(#1108),#896,.F.);
#3571=ADVANCED_FACE('',(#1109),#897,.F.);
#3572=ADVANCED_FACE('',(#1110),#898,.F.);
#3573=ADVANCED_FACE('',(#1111),#899,.F.);
#3574=ADVANCED_FACE('',(#1112),#900,.F.);
#3575=ADVANCED_FACE('',(#1113),#901,.T.);
#3576=ADVANCED_FACE('',(#1114),#902,.F.);
#3577=ADVANCED_FACE('',(#1115),#903,.F.);
#3578=ADVANCED_FACE('',(#1116),#415,.F.);
#3579=ADVANCED_FACE('',(#1117),#904,.F.);
#3580=ADVANCED_FACE('',(#1118),#195,.F.);
#3581=ADVANCED_FACE('',(#1119,#127),#416,.T.);
#3582=ADVANCED_FACE('',(#1120,#128),#417,.F.);
#3583=ADVANCED_FACE('',(#1121),#418,.T.);
#3584=ADVANCED_FACE('',(#1122),#196,.F.);
#3585=ADVANCED_FACE('',(#1123,#129),#419,.T.);
#3586=ADVANCED_FACE('',(#1124,#130),#420,.T.);
#3587=ADVANCED_FACE('',(#1125,#131),#421,.F.);
#3655=CLOSED_SHELL('',(#3565,#3566,#3567,#3568,#3569,#3570,#3571,#3572,
#3573,#3574,#3575,#3576,#3577,#3578,#3579,#3580,#3581,#3582,#3583,#3584,
#3585,#3586,#3587));
#3932=AXIS2_PLACEMENT_3D('',#19351,#4525,#4526);
#3933=AXIS2_PLACEMENT_3D('',#19352,#4527,#4528);
#3934=AXIS2_PLACEMENT_3D('',#19361,#4530,#4531);
#3935=AXIS2_PLACEMENT_3D('',#19373,#4533,#4534);
#3936=AXIS2_PLACEMENT_3D('',#19427,#4536,#4537);
#3937=AXIS2_PLACEMENT_3D('',#19481,#4539,#4540);
#3938=AXIS2_PLACEMENT_3D('',#19514,#4543,#4544);
#3939=AXIS2_PLACEMENT_3D('',#19519,#4546,#4547);
#3940=AXIS2_PLACEMENT_3D('',#19548,#4548,#4549);
#3941=AXIS2_PLACEMENT_3D('',#19582,#4552,#4553);
#3942=AXIS2_PLACEMENT_3D('',#19619,#4554,#4555);
#3943=AXIS2_PLACEMENT_3D('',#19699,#4557,#4558);
#3944=AXIS2_PLACEMENT_3D('',#19725,#4561,#4562);
#3945=AXIS2_PLACEMENT_3D('',#19746,#4563,#4564);
#3946=AXIS2_PLACEMENT_3D('',#19748,#4565,#4566);
#3947=AXIS2_PLACEMENT_3D('',#19751,#4568,#4569);
#3948=AXIS2_PLACEMENT_3D('',#19752,#4570,#4571);
#3949=AXIS2_PLACEMENT_3D('',#19754,#4572,#4573);
#3950=AXIS2_PLACEMENT_3D('',#19757,#4575,#4576);
#3951=AXIS2_PLACEMENT_3D('',#19758,#4577,#4578);
#3952=AXIS2_PLACEMENT_3D('',#19760,#4579,#4580);
#3953=AXIS2_PLACEMENT_3D('',#19763,#4582,#4583);
#3954=AXIS2_PLACEMENT_3D('',#19764,#4584,#4585);
#3955=AXIS2_PLACEMENT_3D('',#19766,#4586,#4587);
#3956=AXIS2_PLACEMENT_3D('',#19769,#4589,#4590);
#3957=AXIS2_PLACEMENT_3D('',#19770,#4591,#4592);
#3958=AXIS2_PLACEMENT_3D('',#19843,#4593,#4594);
#3959=AXIS2_PLACEMENT_3D('',#19846,#4597,#4598);
#3960=AXIS2_PLACEMENT_3D('',#20102,#4600,#4601);
#3961=AXIS2_PLACEMENT_3D('',#20103,#4602,#4603);
#3962=AXIS2_PLACEMENT_3D('',#20104,#4604,#4605);
#3963=AXIS2_PLACEMENT_3D('',#20296,#4607,#4608);
#3964=AXIS2_PLACEMENT_3D('',#20297,#4609,#4610);
#3965=AXIS2_PLACEMENT_3D('',#20298,#4611,#4612);
#4525=DIRECTION('axis',(0.,0.,1.));
#4526=DIRECTION('refdir',(1.,0.,0.));
#4527=DIRECTION('center_axis',(-1.14604935876865E-29,1.,6.74466494129217E-15));
#4528=DIRECTION('ref_axis',(1.,0.,1.79134021914735E-15));
#4529=DIRECTION('',(-1.14604935876865E-29,1.,6.74466494129217E-15));
#4530=DIRECTION('center_axis',(0.,-1.,0.));
#4531=DIRECTION('ref_axis',(1.,0.,1.79134021914735E-15));
#4532=DIRECTION('',(-3.46872215696891E-7,0.999999999999934,1.12705778808245E-7));
#4533=DIRECTION('center_axis',(-1.14604935876865E-29,1.,6.74466494129217E-15));
#4534=DIRECTION('ref_axis',(1.,0.,1.79134021914735E-15));
#4535=DIRECTION('',(-1.14604935876865E-29,1.,6.74466494129217E-15));
#4536=DIRECTION('center_axis',(-1.14604935876865E-29,1.,6.74466494129217E-15));
#4537=DIRECTION('ref_axis',(1.,0.,1.79134021914735E-15));
#4538=DIRECTION('',(-1.14604935876865E-29,1.,6.74466494129217E-15));
#4539=DIRECTION('center_axis',(-1.14604935876865E-29,1.,6.74466494129217E-15));
#4540=DIRECTION('ref_axis',(1.,0.,1.79134021914735E-15));
#4541=DIRECTION('',(-1.14604935876865E-29,1.,6.74466494129217E-15));
#4542=DIRECTION('',(0.,-1.,-3.46944695195361E-16));
#4543=DIRECTION('center_axis',(0.,-1.,0.));
#4544=DIRECTION('ref_axis',(0.,0.,-1.));
#4545=DIRECTION('',(0.,-1.,0.));
#4546=DIRECTION('center_axis',(0.,1.,0.));
#4547=DIRECTION('ref_axis',(0.,0.,1.));
#4548=DIRECTION('center_axis',(0.,-1.,0.));
#4549=DIRECTION('ref_axis',(0.,0.,-1.));
#4550=DIRECTION('',(0.,-1.,0.));
#4551=DIRECTION('',(0.,1.,0.));
#4552=DIRECTION('center_axis',(0.,1.,0.));
#4553=DIRECTION('ref_axis',(0.,0.,1.));
#4554=DIRECTION('center_axis',(0.,-1.,0.));
#4555=DIRECTION('ref_axis',(0.,0.,-1.));
#4556=DIRECTION('',(0.,-1.,0.));
#4557=DIRECTION('center_axis',(0.,-1.,0.));
#4558=DIRECTION('ref_axis',(0.,0.,-1.));
#4559=DIRECTION('',(0.,-1.,0.));
#4560=DIRECTION('',(3.46872213130258E-7,-0.999999999999933,-1.1270548577469E-7));
#4561=DIRECTION('center_axis',(0.,1.,0.));
#4562=DIRECTION('ref_axis',(0.,0.,1.));
#4563=DIRECTION('center_axis',(0.,1.,0.));
#4564=DIRECTION('ref_axis',(0.,0.,1.));
#4565=DIRECTION('center_axis',(0.,1.,0.));
#4566=DIRECTION('ref_axis',(0.,0.,1.));
#4567=DIRECTION('',(0.,1.,0.));
#4568=DIRECTION('center_axis',(0.,1.,0.));
#4569=DIRECTION('ref_axis',(0.,0.,1.));
#4570=DIRECTION('center_axis',(0.,1.,0.));
#4571=DIRECTION('ref_axis',(0.,0.,1.));
#4572=DIRECTION('center_axis',(0.,1.,0.));
#4573=DIRECTION('ref_axis',(0.,0.,1.));
#4574=DIRECTION('',(0.,1.,0.));
#4575=DIRECTION('center_axis',(0.,1.,0.));
#4576=DIRECTION('ref_axis',(0.,0.,1.));
#4577=DIRECTION('center_axis',(0.,-1.,0.));
#4578=DIRECTION('ref_axis',(0.,0.,-1.));
#4579=DIRECTION('center_axis',(0.,1.,0.));
#4580=DIRECTION('ref_axis',(0.,0.,1.));
#4581=DIRECTION('',(0.,1.,0.));
#4582=DIRECTION('center_axis',(0.,1.,0.));
#4583=DIRECTION('ref_axis',(0.,0.,1.));
#4584=DIRECTION('center_axis',(0.,-1.,0.));
#4585=DIRECTION('ref_axis',(0.,0.,-1.));
#4586=DIRECTION('center_axis',(0.,1.,0.));
#4587=DIRECTION('ref_axis',(0.,0.,1.));
#4588=DIRECTION('',(0.,-1.,0.));
#4589=DIRECTION('center_axis',(0.,1.,0.));
#4590=DIRECTION('ref_axis',(0.,0.,1.));
#4591=DIRECTION('center_axis',(0.,-1.,0.));
#4592=DIRECTION('ref_axis',(0.,0.,-1.));
#4593=DIRECTION('center_axis',(-0.951056619716827,-3.64722989082937E-7,
0.30901667607537));
#4594=DIRECTION('ref_axis',(0.309016676075391,1.57739547043686E-23,0.95105661971689));
#4595=DIRECTION('',(-0.309016676075391,0.,-0.95105661971689));
#4596=DIRECTION('',(-0.267616460838902,0.500000023942052,-0.82363912361301));
#4597=DIRECTION('center_axis',(-1.14604935876865E-29,1.,6.74466494129217E-15));
#4598=DIRECTION('ref_axis',(1.,0.,1.79134021914735E-15));
#4599=DIRECTION('',(-0.866025403784441,-0.499999999999996,0.));
#4600=DIRECTION('center_axis',(0.,1.,0.));
#4601=DIRECTION('ref_axis',(0.,0.,1.));
#4602=DIRECTION('center_axis',(0.,1.,0.));
#4603=DIRECTION('ref_axis',(0.,0.,1.));
#4604=DIRECTION('center_axis',(0.,0.,1.));
#4605=DIRECTION('ref_axis',(1.,0.,0.));
#4606=DIRECTION('',(0.866025403784441,-0.499999999999996,1.38777878684589E-16));
#4607=DIRECTION('center_axis',(0.,1.,0.));
#4608=DIRECTION('ref_axis',(0.,0.,1.));
#4609=DIRECTION('center_axis',(0.,1.,0.));
#4610=DIRECTION('ref_axis',(0.,0.,1.));
#4611=DIRECTION('center_axis',(0.,1.,0.));
#4612=DIRECTION('ref_axis',(0.,0.,1.));
#19351=CARTESIAN_POINT('',(0.,0.,0.));
#19352=CARTESIAN_POINT('Origin',(-4.44089209850063E-14,2.18749999317203,
-8.4502213867173E-14));
#19353=CARTESIAN_POINT('',(-47.293670625,19.062499993172,-2.74087067386922E-14));
#19354=CARTESIAN_POINT('',(-47.293670625,20.312499993172,-2.29764507158874E-14));
#19355=CARTESIAN_POINT('',(-47.2936706250001,2.18749999317203,-1.6342946393376E-13));
#19356=CARTESIAN_POINT('',(-44.6588684919845,20.58,15.5652416043447));
#19357=CARTESIAN_POINT('Ctrl Pts',(-47.293670625,20.312499993172,-4.77048955893622E-15));
#19358=CARTESIAN_POINT('Ctrl Pts',(-47.293670625,20.4441128906546,8.00562351734399));
#19359=CARTESIAN_POINT('Ctrl Pts',(-44.6588684919845,20.58,15.5652416043447));
#19360=CARTESIAN_POINT('',(14.6145423619412,20.58,44.9789554429287));
#19361=CARTESIAN_POINT('Origin',(-4.44089209850065E-14,20.58,3.95490361115957E-14));
#19362=CARTESIAN_POINT('',(14.6145423715095,20.5629604749638,44.9789554528196));
#19363=CARTESIAN_POINT('',(14.6145423672912,20.5629605363188,44.9789554411892));
#19364=CARTESIAN_POINT('Ctrl Pts',(-47.293670625,19.062499993172,-5.20417042793042E-15));
#19365=CARTESIAN_POINT('Ctrl Pts',(-47.293670625,19.2708333265054,12.6723008510722));
#19366=CARTESIAN_POINT('Ctrl Pts',(-40.9575201994638,19.4791666598387,23.6468353125));
#19367=CARTESIAN_POINT('Ctrl Pts',(-34.6213697739277,19.687499993172,34.6213697739277));
#19368=CARTESIAN_POINT('Ctrl Pts',(-23.6468353125,19.8958333265054,40.9575201994639));
#19369=CARTESIAN_POINT('Ctrl Pts',(-12.6723008510723,20.1041666598387,47.293670625));
#19370=CARTESIAN_POINT('Ctrl Pts',(-2.77555756156289E-14,20.312499993172,
47.293670625));
#19371=CARTESIAN_POINT('Ctrl Pts',(7.4905755366668,20.4356454731033,47.293670625));
#19372=CARTESIAN_POINT('Ctrl Pts',(14.6145423683093,20.5629604365775,44.9789554408594));
#19373=CARTESIAN_POINT('Origin',(-4.44089209850063E-14,2.18749999317203,
-8.4502213867173E-14));
#19374=CARTESIAN_POINT('',(-47.293670625,14.062499993172,-4.42703690919226E-14));
#19375=CARTESIAN_POINT('',(-47.293670625,15.312499993172,-3.98381130691179E-14));
#19376=CARTESIAN_POINT('',(-47.2936706250001,2.18749999317203,-1.6342946393376E-13));
#19377=CARTESIAN_POINT('Ctrl Pts',(-47.293670625,15.312499993172,-4.77048955893622E-15));
#19378=CARTESIAN_POINT('Ctrl Pts',(-47.293670625,15.5208333265054,12.6723008510722));
#19379=CARTESIAN_POINT('Ctrl Pts',(-40.9575201994638,15.7291666598387,23.6468353125));
#19380=CARTESIAN_POINT('Ctrl Pts',(-34.6213697739277,15.937499993172,34.6213697739277));
#19381=CARTESIAN_POINT('Ctrl Pts',(-23.6468353125,16.1458333265054,40.9575201994638));
#19382=CARTESIAN_POINT('Ctrl Pts',(-12.6723008510723,16.3541666598387,47.293670625));
#19383=CARTESIAN_POINT('Ctrl Pts',(-2.77555756156289E-14,16.562499993172,
47.293670625));
#19384=CARTESIAN_POINT('Ctrl Pts',(12.6723008510722,16.7708333265054,47.293670625));
#19385=CARTESIAN_POINT('Ctrl Pts',(23.6468353125,16.9791666598387,40.9575201994639));
#19386=CARTESIAN_POINT('Ctrl Pts',(34.6213697739277,17.187499993172,34.6213697739278));
#19387=CARTESIAN_POINT('Ctrl Pts',(40.9575201994639,17.3958333265054,23.6468353125));
#19388=CARTESIAN_POINT('Ctrl Pts',(47.293670625,17.6041666598387,12.6723008510723));
#19389=CARTESIAN_POINT('Ctrl Pts',(47.293670625,17.812499993172,4.33680868994202E-16));
#19390=CARTESIAN_POINT('Ctrl Pts',(47.293670625,18.0208333265054,-12.6723008510723));
#19391=CARTESIAN_POINT('Ctrl Pts',(40.9575201994639,18.2291666598387,-23.6468353125));
#19392=CARTESIAN_POINT('Ctrl Pts',(34.6213697739278,18.437499993172,-34.6213697739277));
#19393=CARTESIAN_POINT('Ctrl Pts',(23.6468353125,18.6458333265054,-40.9575201994639));
#19394=CARTESIAN_POINT('Ctrl Pts',(12.6723008510723,18.8541666598387,-47.293670625));
#19395=CARTESIAN_POINT('Ctrl Pts',(0.,19.062499993172,-47.293670625));
#19396=CARTESIAN_POINT('Ctrl Pts',(-12.6723008510723,19.2708333265054,-47.293670625));
#19397=CARTESIAN_POINT('Ctrl Pts',(-23.6468353125,19.4791666598387,-40.9575201994639));
#19398=CARTESIAN_POINT('Ctrl Pts',(-34.6213697739277,19.687499993172,-34.6213697739277));
#19399=CARTESIAN_POINT('Ctrl Pts',(-40.9575201994638,19.8958333265054,-23.6468353125));
#19400=CARTESIAN_POINT('Ctrl Pts',(-47.293670625,20.1041666598387,-12.6723008510723));
#19401=CARTESIAN_POINT('Ctrl Pts',(-47.293670625,20.312499993172,-4.77048955893622E-15));
#19402=CARTESIAN_POINT('Ctrl Pts',(-47.293670625,14.062499993172,-5.20417042793042E-15));
#19403=CARTESIAN_POINT('Ctrl Pts',(-47.293670625,14.2708333265054,12.6723008510722));
#19404=CARTESIAN_POINT('Ctrl Pts',(-40.9575201994638,14.4791666598387,23.6468353125));
#19405=CARTESIAN_POINT('Ctrl Pts',(-34.6213697739277,14.687499993172,34.6213697739277));
#19406=CARTESIAN_POINT('Ctrl Pts',(-23.6468353125,14.8958333265054,40.9575201994639));
#19407=CARTESIAN_POINT('Ctrl Pts',(-12.6723008510723,15.1041666598387,47.293670625));
#19408=CARTESIAN_POINT('Ctrl Pts',(-2.77555756156289E-14,15.312499993172,
47.293670625));
#19409=CARTESIAN_POINT('Ctrl Pts',(12.6723008510722,15.5208333265054,47.293670625));
#19410=CARTESIAN_POINT('Ctrl Pts',(23.6468353125,15.7291666598387,40.9575201994639));
#19411=CARTESIAN_POINT('Ctrl Pts',(34.6213697739277,15.937499993172,34.6213697739278));
#19412=CARTESIAN_POINT('Ctrl Pts',(40.9575201994639,16.1458333265054,23.6468353125));
#19413=CARTESIAN_POINT('Ctrl Pts',(47.293670625,16.3541666598387,12.6723008510723));
#19414=CARTESIAN_POINT('Ctrl Pts',(47.293670625,16.562499993172,0.));
#19415=CARTESIAN_POINT('Ctrl Pts',(47.293670625,16.7708333265054,-12.6723008510723));
#19416=CARTESIAN_POINT('Ctrl Pts',(40.9575201994639,16.9791666598387,-23.6468353125));
#19417=CARTESIAN_POINT('Ctrl Pts',(34.6213697739278,17.187499993172,-34.6213697739277));
#19418=CARTESIAN_POINT('Ctrl Pts',(23.6468353125,17.3958333265054,-40.9575201994639));
#19419=CARTESIAN_POINT('Ctrl Pts',(12.6723008510723,17.6041666598387,-47.293670625));
#19420=CARTESIAN_POINT('Ctrl Pts',(0.,17.812499993172,-47.293670625));
#19421=CARTESIAN_POINT('Ctrl Pts',(-12.6723008510723,18.0208333265054,-47.293670625));
#19422=CARTESIAN_POINT('Ctrl Pts',(-23.6468353125,18.2291666598387,-40.9575201994639));
#19423=CARTESIAN_POINT('Ctrl Pts',(-34.6213697739277,18.437499993172,-34.6213697739278));
#19424=CARTESIAN_POINT('Ctrl Pts',(-40.9575201994638,18.6458333265054,-23.6468353125));
#19425=CARTESIAN_POINT('Ctrl Pts',(-47.293670625,18.8541666598387,-12.6723008510723));
#19426=CARTESIAN_POINT('Ctrl Pts',(-47.293670625,19.062499993172,-5.20417042793042E-15));
#19427=CARTESIAN_POINT('Origin',(-4.44089209850063E-14,2.18749999317203,
-8.4502213867173E-14));
#19428=CARTESIAN_POINT('',(-47.293670625,9.06249999317203,-6.11320314451531E-14));
#19429=CARTESIAN_POINT('',(-47.293670625,10.312499993172,-5.66997754223483E-14));
#19430=CARTESIAN_POINT('',(-47.2936706250001,2.18749999317203,-1.6342946393376E-13));
#19431=CARTESIAN_POINT('Ctrl Pts',(-47.293670625,10.312499993172,-4.77048955893622E-15));
#19432=CARTESIAN_POINT('Ctrl Pts',(-47.293670625,10.5208333265054,12.6723008510722));
#19433=CARTESIAN_POINT('Ctrl Pts',(-40.9575201994638,10.7291666598387,23.6468353125));
#19434=CARTESIAN_POINT('Ctrl Pts',(-34.6213697739277,10.937499993172,34.6213697739277));
#19435=CARTESIAN_POINT('Ctrl Pts',(-23.6468353125,11.1458333265054,40.9575201994638));
#19436=CARTESIAN_POINT('Ctrl Pts',(-12.6723008510723,11.3541666598387,47.293670625));
#19437=CARTESIAN_POINT('Ctrl Pts',(-2.77555756156289E-14,11.562499993172,
47.293670625));
#19438=CARTESIAN_POINT('Ctrl Pts',(12.6723008510722,11.7708333265054,47.293670625));
#19439=CARTESIAN_POINT('Ctrl Pts',(23.6468353125,11.9791666598387,40.9575201994639));
#19440=CARTESIAN_POINT('Ctrl Pts',(34.6213697739277,12.187499993172,34.6213697739278));
#19441=CARTESIAN_POINT('Ctrl Pts',(40.9575201994639,12.3958333265054,23.6468353125));
#19442=CARTESIAN_POINT('Ctrl Pts',(47.293670625,12.6041666598387,12.6723008510723));
#19443=CARTESIAN_POINT('Ctrl Pts',(47.293670625,12.812499993172,4.33680868994202E-16));
#19444=CARTESIAN_POINT('Ctrl Pts',(47.293670625,13.0208333265054,-12.6723008510723));
#19445=CARTESIAN_POINT('Ctrl Pts',(40.9575201994639,13.2291666598387,-23.6468353125));
#19446=CARTESIAN_POINT('Ctrl Pts',(34.6213697739278,13.437499993172,-34.6213697739277));
#19447=CARTESIAN_POINT('Ctrl Pts',(23.6468353125,13.6458333265054,-40.9575201994639));
#19448=CARTESIAN_POINT('Ctrl Pts',(12.6723008510723,13.8541666598387,-47.293670625));
#19449=CARTESIAN_POINT('Ctrl Pts',(0.,14.062499993172,-47.293670625));
#19450=CARTESIAN_POINT('Ctrl Pts',(-12.6723008510723,14.2708333265054,-47.293670625));
#19451=CARTESIAN_POINT('Ctrl Pts',(-23.6468353125,14.4791666598387,-40.9575201994639));
#19452=CARTESIAN_POINT('Ctrl Pts',(-34.6213697739277,14.687499993172,-34.6213697739277));
#19453=CARTESIAN_POINT('Ctrl Pts',(-40.9575201994638,14.8958333265054,-23.6468353125));
#19454=CARTESIAN_POINT('Ctrl Pts',(-47.293670625,15.1041666598387,-12.6723008510723));
#19455=CARTESIAN_POINT('Ctrl Pts',(-47.293670625,15.312499993172,-4.77048955893622E-15));
#19456=CARTESIAN_POINT('Ctrl Pts',(-47.293670625,9.06249999317203,-5.20417042793042E-15));
#19457=CARTESIAN_POINT('Ctrl Pts',(-47.293670625,9.27083332650536,12.6723008510722));
#19458=CARTESIAN_POINT('Ctrl Pts',(-40.9575201994638,9.4791666598387,23.6468353125));
#19459=CARTESIAN_POINT('Ctrl Pts',(-34.6213697739277,9.68749999317203,34.6213697739277));
#19460=CARTESIAN_POINT('Ctrl Pts',(-23.6468353125,9.89583332650536,40.9575201994639));
#19461=CARTESIAN_POINT('Ctrl Pts',(-12.6723008510723,10.1041666598387,47.293670625));
#19462=CARTESIAN_POINT('Ctrl Pts',(-2.77555756156289E-14,10.312499993172,
47.293670625));
#19463=CARTESIAN_POINT('Ctrl Pts',(12.6723008510722,10.5208333265054,47.293670625));
#19464=CARTESIAN_POINT('Ctrl Pts',(23.6468353125,10.7291666598387,40.9575201994639));
#19465=CARTESIAN_POINT('Ctrl Pts',(34.6213697739277,10.937499993172,34.6213697739278));
#19466=CARTESIAN_POINT('Ctrl Pts',(40.9575201994639,11.1458333265054,23.6468353125));
#19467=CARTESIAN_POINT('Ctrl Pts',(47.293670625,11.3541666598387,12.6723008510723));
#19468=CARTESIAN_POINT('Ctrl Pts',(47.293670625,11.562499993172,0.));
#19469=CARTESIAN_POINT('Ctrl Pts',(47.293670625,11.7708333265054,-12.6723008510723));
#19470=CARTESIAN_POINT('Ctrl Pts',(40.9575201994639,11.9791666598387,-23.6468353125));
#19471=CARTESIAN_POINT('Ctrl Pts',(34.6213697739278,12.187499993172,-34.6213697739277));
#19472=CARTESIAN_POINT('Ctrl Pts',(23.6468353125,12.3958333265054,-40.9575201994639));
#19473=CARTESIAN_POINT('Ctrl Pts',(12.6723008510723,12.6041666598387,-47.293670625));
#19474=CARTESIAN_POINT('Ctrl Pts',(0.,12.812499993172,-47.293670625));
#19475=CARTESIAN_POINT('Ctrl Pts',(-12.6723008510723,13.0208333265054,-47.293670625));
#19476=CARTESIAN_POINT('Ctrl Pts',(-23.6468353125,13.2291666598387,-40.9575201994639));
#19477=CARTESIAN_POINT('Ctrl Pts',(-34.6213697739277,13.437499993172,-34.6213697739278));
#19478=CARTESIAN_POINT('Ctrl Pts',(-40.9575201994638,13.6458333265054,-23.6468353125));
#19479=CARTESIAN_POINT('Ctrl Pts',(-47.293670625,13.8541666598387,-12.6723008510723));
#19480=CARTESIAN_POINT('Ctrl Pts',(-47.293670625,14.062499993172,-5.20417042793042E-15));
#19481=CARTESIAN_POINT('Origin',(-4.44089209850063E-14,2.18749999317203,
-8.4502213867173E-14));
#19482=CARTESIAN_POINT('',(-47.293670625,4.06249999317204,-7.79936937983835E-14));
#19483=CARTESIAN_POINT('',(-47.293670625,5.31249999317204,-7.35614377755788E-14));
#19484=CARTESIAN_POINT('',(-47.2936706250001,2.18749999317203,-1.6342946393376E-13));
#19485=CARTESIAN_POINT('',(47.293670625,1.56249999317203,0.));
#19486=CARTESIAN_POINT('Ctrl Pts',(47.293670625,1.56249999317203,0.));
#19487=CARTESIAN_POINT('Ctrl Pts',(47.293670625,1.77083332650536,-12.6723008510723));
#19488=CARTESIAN_POINT('Ctrl Pts',(40.9575201994639,1.9791666598387,-23.6468353125));
#19489=CARTESIAN_POINT('Ctrl Pts',(34.6213697739278,2.18749999317203,-34.6213697739277));
#19490=CARTESIAN_POINT('Ctrl Pts',(23.6468353125,2.39583332650536,-40.9575201994639));
#19491=CARTESIAN_POINT('Ctrl Pts',(12.6723008510723,2.6041666598387,-47.293670625));
#19492=CARTESIAN_POINT('Ctrl Pts',(0.,2.81249999317203,-47.293670625));
#19493=CARTESIAN_POINT('Ctrl Pts',(-12.6723008510723,3.02083332650537,-47.293670625));
#19494=CARTESIAN_POINT('Ctrl Pts',(-23.6468353125,3.2291666598387,-40.9575201994639));
#19495=CARTESIAN_POINT('Ctrl Pts',(-34.6213697739277,3.43749999317203,-34.6213697739278));
#19496=CARTESIAN_POINT('Ctrl Pts',(-40.9575201994638,3.64583332650537,-23.6468353125));
#19497=CARTESIAN_POINT('Ctrl Pts',(-47.293670625,3.8541666598387,-12.6723008510723));
#19498=CARTESIAN_POINT('Ctrl Pts',(-47.293670625,4.06249999317204,-5.20417042793042E-15));
#19499=CARTESIAN_POINT('',(47.293670625,2.81249999317203,4.33680868994202E-16));
#19500=CARTESIAN_POINT('',(47.293670625,2.81249999317203,4.33680868994202E-16));
#19501=CARTESIAN_POINT('Ctrl Pts',(47.293670625,2.81249999317203,4.33680868994202E-16));
#19502=CARTESIAN_POINT('Ctrl Pts',(47.293670625,3.02083332650537,-12.6723008510723));
#19503=CARTESIAN_POINT('Ctrl Pts',(40.9575201994639,3.2291666598387,-23.6468353125));
#19504=CARTESIAN_POINT('Ctrl Pts',(34.6213697739278,3.43749999317203,-34.6213697739277));
#19505=CARTESIAN_POINT('Ctrl Pts',(23.6468353125,3.64583332650537,-40.9575201994639));
#19506=CARTESIAN_POINT('Ctrl Pts',(12.6723008510723,3.8541666598387,-47.293670625));
#19507=CARTESIAN_POINT('Ctrl Pts',(0.,4.06249999317204,-47.293670625));
#19508=CARTESIAN_POINT('Ctrl Pts',(-12.6723008510723,4.27083332650536,-47.293670625));
#19509=CARTESIAN_POINT('Ctrl Pts',(-23.6468353125,4.4791666598387,-40.9575201994639));
#19510=CARTESIAN_POINT('Ctrl Pts',(-34.6213697739277,4.68749999317204,-34.6213697739277));
#19511=CARTESIAN_POINT('Ctrl Pts',(-40.9575201994638,4.89583332650537,-23.6468353125));
#19512=CARTESIAN_POINT('Ctrl Pts',(-47.293670625,5.1041666598387,-12.6723008510723));
#19513=CARTESIAN_POINT('Ctrl Pts',(-47.293670625,5.31249999317204,-4.77048955893622E-15));
#19514=CARTESIAN_POINT('Origin',(0.,30.,0.));
#19515=CARTESIAN_POINT('',(-3.61672851018096E-15,3.75,50.));
#19516=CARTESIAN_POINT('',(-6.12323399573677E-15,0.,50.));
#19517=CARTESIAN_POINT('',(-6.12323399573677E-15,30.,50.));
#19518=CARTESIAN_POINT('',(50.,0.,4.33680868994202E-16));
#19519=CARTESIAN_POINT('Origin',(0.,0.,0.));
#19520=CARTESIAN_POINT('Ctrl Pts',(50.,1.06165076729781E-14,-2.22044604925031E-15));
#19521=CARTESIAN_POINT('Ctrl Pts',(50.,0.0675815458886919,-4.34602095458794));
#19522=CARTESIAN_POINT('Ctrl Pts',(49.433363177975,0.137236267109327,-8.67353338775704));
#19523=CARTESIAN_POINT('Ctrl Pts',(47.1953230212392,0.277178851018911,-17.0732528980021));
#19524=CARTESIAN_POINT('Ctrl Pts',(45.5332330036253,0.346871852511727,-21.1097012523794));
#19525=CARTESIAN_POINT('Ctrl Pts',(40.1317492627809,0.515793945868729,-30.5253872857993));
#19526=CARTESIAN_POINT('Ctrl Pts',(35.8219475848477,0.621158082158269,-35.4844500978245));
#19527=CARTESIAN_POINT('Ctrl Pts',(25.5795028430515,0.828373107047328,-43.4450365132807));
#19528=CARTESIAN_POINT('Ctrl Pts',(19.7547036395998,0.927746124936861,-46.3846276563406));
#19529=CARTESIAN_POINT('Ctrl Pts',(7.27375715639306,1.1364474793245,-49.8934263074991));
#19530=CARTESIAN_POINT('Ctrl Pts',(0.731992466642528,1.2368859786089,-50.4155320575528));
#19531=CARTESIAN_POINT('Ctrl Pts',(-12.2694666320475,1.4453065174627,-48.9167086614796));
#19532=CARTESIAN_POINT('Ctrl Pts',(-18.5997310439367,1.55224307809009,-46.8768025214219));
#19533=CARTESIAN_POINT('Ctrl Pts',(-30.0299904422847,1.75654526614157,-40.5025862073931));
#19534=CARTESIAN_POINT('Ctrl Pts',(-35.036045408383,1.86107507457517,-36.2592957566779));
#19535=CARTESIAN_POINT('Ctrl Pts',(-43.120111853279,2.06848140107261,-26.1235259446925));
#19536=CARTESIAN_POINT('Ctrl Pts',(-46.1326953039639,2.16765558228902,-20.3360992301171));
#19537=CARTESIAN_POINT('Ctrl Pts',(-49.8001432688674,2.37642657857554,-7.89318418467289));
#19538=CARTESIAN_POINT('Ctrl Pts',(-50.403689005381,2.47731150480502,-1.35087920859845));
#19539=CARTESIAN_POINT('Ctrl Pts',(-49.0628121307921,2.68532756322191,11.6668902834284));
#19540=CARTESIAN_POINT('Ctrl Pts',(-47.1039105257039,2.79218578597068,18.0138220579311));
#19541=CARTESIAN_POINT('Ctrl Pts',(-40.881726186314,2.99688303055821,29.5102235202591));
#19542=CARTESIAN_POINT('Ctrl Pts',(-36.7076021277602,3.10060669623969,34.5647456017332));
#19543=CARTESIAN_POINT('Ctrl Pts',(-26.6829381859637,3.30819972311771,42.7763188165426));
#19544=CARTESIAN_POINT('Ctrl Pts',(-20.9345141514266,3.40723200021609,45.8643504967883));
#19545=CARTESIAN_POINT('Ctrl Pts',(-9.96972190006956,3.59185030232342,49.2515812260447));
#19546=CARTESIAN_POINT('Ctrl Pts',(-4.99455109538804,3.67233367312923,50.));
#19547=CARTESIAN_POINT('Ctrl Pts',(1.11022302462516E-15,3.75000000000001,
50.));
#19548=CARTESIAN_POINT('Origin',(0.,30.,0.));
#19549=CARTESIAN_POINT('',(-1.63842932933703E-14,8.75,50.));
#19550=CARTESIAN_POINT('',(2.8024627691636E-14,8.12499998634407,50.));
#19551=CARTESIAN_POINT('',(-6.12323399573677E-15,30.,50.));
#19552=CARTESIAN_POINT('',(50.,4.37499998634407,4.33680868994202E-16));
#19553=CARTESIAN_POINT('Ctrl Pts',(3.77475828372553E-14,8.12499998634407,
50.));
#19554=CARTESIAN_POINT('Ctrl Pts',(-6.29656683951167,8.02708703901777,50.));
#19555=CARTESIAN_POINT('Ctrl Pts',(-12.5395378026787,7.92505148761976,48.8105524892163));
#19556=CARTESIAN_POINT('Ctrl Pts',(-24.428748973416,7.72056704948577,44.1054274881654));
#19557=CARTESIAN_POINT('Ctrl Pts',(-29.9370959070449,7.62102578272423,40.568739744262));
#19558=CARTESIAN_POINT('Ctrl Pts',(-39.2829518076402,7.4125611305386,31.6017896070106));
#19559=CARTESIAN_POINT('Ctrl Pts',(-43.036824942223,7.31238179776275,26.2612876234044));
#19560=CARTESIAN_POINT('Ctrl Pts',(-48.3273553137792,7.10574897519395,14.3907774590969));
#19561=CARTESIAN_POINT('Ctrl Pts',(-49.791594591191,6.99971009509526,7.96399144170724));
#19562=CARTESIAN_POINT('Ctrl Pts',(-50.1681486104848,6.79458070879849,-5.12653202942374));
#19563=CARTESIAN_POINT('Ctrl Pts',(-49.0619331605251,6.68971160553214,-11.6641350292155));
#19564=CARTESIAN_POINT('Ctrl Pts',(-44.4171209681097,6.48077343574223,-23.8559166804422));
#19565=CARTESIAN_POINT('Ctrl Pts',(-40.9550834065452,6.38147848262782,-29.4052106806457));
#19566=CARTESIAN_POINT('Ctrl Pts',(-32.113466366765,6.17312980425173,-38.8662118322004));
#19567=CARTESIAN_POINT('Ctrl Pts',(-26.820282375283,6.07251482308326,-42.6910956804875));
#19568=CARTESIAN_POINT('Ctrl Pts',(-15.009584552541,5.86615268861856,-48.1398836046983));
#19569=CARTESIAN_POINT('Ctrl Pts',(-8.59369004350663,5.75993421526962,-49.6878729247248));
#19570=CARTESIAN_POINT('Ctrl Pts',(4.48774492525712,5.55426543933499,-50.2277992097));
#19571=CARTESIAN_POINT('Ctrl Pts',(11.0271640436078,5.45022299225461,-49.2074578926806));
#19572=CARTESIAN_POINT('Ctrl Pts',(23.2638995025692,5.24128050504109,-44.729379413062));
#19573=CARTESIAN_POINT('Ctrl Pts',(28.8548134450474,5.14217116635957,-41.3439967022577));
#19574=CARTESIAN_POINT('Ctrl Pts',(38.433121503277,4.93395386608903,-32.6312276229427));
#19575=CARTESIAN_POINT('Ctrl Pts',(42.3304633933119,4.83282603182798,-27.3867424586433));
#19576=CARTESIAN_POINT('Ctrl Pts',(46.7247122573551,4.67141859868476,-18.1844199659609));
#19577=CARTESIAN_POINT('Ctrl Pts',(47.949072379614,4.61142813276804,-14.6546310169365));
#19578=CARTESIAN_POINT('Ctrl Pts',(49.5874843271383,4.49186567045974,-7.404842522204));
#19579=CARTESIAN_POINT('Ctrl Pts',(50.,4.43266281444172,-3.7081699732958));
#19580=CARTESIAN_POINT('Ctrl Pts',(50.,4.37499998634406,-1.11022302462516E-15));
#19581=CARTESIAN_POINT('',(50.,2.18749999317203,4.33680868994202E-16));
#19582=CARTESIAN_POINT('Origin',(0.,0.,0.));
#19583=CARTESIAN_POINT('Ctrl Pts',(-1.38777878078145E-15,3.75000000000001,
50.));
#19584=CARTESIAN_POINT('Ctrl Pts',(1.50002951166462,3.77332577645995,50.));
#19585=CARTESIAN_POINT('Ctrl Pts',(3.00179837118478,3.79695985428445,49.9324990070492));
#19586=CARTESIAN_POINT('Ctrl Pts',(11.0440849325066,3.9250477770621,49.2056195962975));
#19587=CARTESIAN_POINT('Ctrl Pts',(17.4071452363091,4.0318085869817,47.3302895610126));
#19588=CARTESIAN_POINT('Ctrl Pts',(28.9703187695284,4.23689013305346,41.2650696264942));
#19589=CARTESIAN_POINT('Ctrl Pts',(34.0743240006798,4.33984944424209,37.162163128162));
#19590=CARTESIAN_POINT('Ctrl Pts',(42.4162332551277,4.54762178810859,27.2520829284582));
#19591=CARTESIAN_POINT('Ctrl Pts',(45.5814688037948,4.64657621006581,21.5439667179538));
#19592=CARTESIAN_POINT('Ctrl Pts',(49.5807884827107,4.85545523193025,9.18302954234058));
#19593=CARTESIAN_POINT('Ctrl Pts',(50.3548312508471,4.95745741831768,2.64074335025333));
#19594=CARTESIAN_POINT('Ctrl Pts',(49.3431424035077,5.16456855488943,-10.4070382692032));
#19595=CARTESIAN_POINT('Ctrl Pts',(47.5531367195831,5.27121261121499,-16.7854529965516));
#19596=CARTESIAN_POINT('Ctrl Pts',(41.6483204537289,5.47666231002944,-28.4152816584745));
#19597=CARTESIAN_POINT('Ctrl Pts',(37.6180020049751,5.57891128315246,-33.5692881184128));
#19598=CARTESIAN_POINT('Ctrl Pts',(27.8249007712785,5.78685301485799,-42.0430563993917));
#19599=CARTESIAN_POINT('Ctrl Pts',(22.1580244614444,5.88579837872905,-45.286483980451));
#19600=CARTESIAN_POINT('Ctrl Pts',(9.8403808718465,6.09471262938967,-49.4558324330969));
#19601=CARTESIAN_POINT('Ctrl Pts',(3.2987214372498,6.19738209975368,-50.3173000552676));
#19602=CARTESIAN_POINT('Ctrl Pts',(-9.76230561520494,6.40399928058008,-49.4735932157222));
#19603=CARTESIAN_POINT('Ctrl Pts',(-16.155095216762,6.51050773208155,-47.7697804504798));
#19604=CARTESIAN_POINT('Ctrl Pts',(-27.8507188284245,6.7163046564155,-42.0271801552601));
#19605=CARTESIAN_POINT('Ctrl Pts',(-33.0547271997935,6.81790741632008,-38.0700878384781));
#19606=CARTESIAN_POINT('Ctrl Pts',(-41.6605133560118,7.02600643206108,-28.3951876913978));
#19607=CARTESIAN_POINT('Ctrl Pts',(-44.9823163989605,7.12501350110592,-22.7700748235208));
#19608=CARTESIAN_POINT('Ctrl Pts',(-49.3221121430825,7.33394910022637,-10.4967295754095));
#19609=CARTESIAN_POINT('Ctrl Pts',(-50.2712713321659,7.43735106074952,-3.95612890853374));
#19610=CARTESIAN_POINT('Ctrl Pts',(-49.5954802301861,7.64345278002998,9.11674282900515));
#19611=CARTESIAN_POINT('Ctrl Pts',(-47.9778112005811,7.74980803904956,15.5227631025264));
#19612=CARTESIAN_POINT('Ctrl Pts',(-42.3975433426475,7.95592734940999,27.2826154977726));
#19613=CARTESIAN_POINT('Ctrl Pts',(-38.5135601479802,8.05695543575843,32.5361107635385));
#19614=CARTESIAN_POINT('Ctrl Pts',(-28.9568652006334,8.26519795013379,41.2727079144305));
#19615=CARTESIAN_POINT('Ctrl Pts',(-23.3736122913173,8.36433646334925,44.6722598314387));
#19616=CARTESIAN_POINT('Ctrl Pts',(-11.7545603061111,8.5628659464166,48.9564434230258));
#19617=CARTESIAN_POINT('Ctrl Pts',(-5.89770451089775,8.65828944632209,50.));
#19618=CARTESIAN_POINT('Ctrl Pts',(-7.7715611723761E-15,8.75,50.));
#19619=CARTESIAN_POINT('Origin',(0.,30.,0.));
#19620=CARTESIAN_POINT('',(-2.42252434047854E-14,13.75,50.));
#19621=CARTESIAN_POINT('',(-4.17184002249354E-15,13.1249999863441,50.));
#19622=CARTESIAN_POINT('',(-6.12323399573677E-15,30.,50.));
#19623=CARTESIAN_POINT('Ctrl Pts',(-5.96744875736022E-15,13.1249999863441,
50.));
#19624=CARTESIAN_POINT('Ctrl Pts',(-0.612619827520453,13.1154736183356,
50.));
#19625=CARTESIAN_POINT('Ctrl Pts',(-1.22568533661716,13.1058934073382,49.9887409889087));
#19626=CARTESIAN_POINT('Ctrl Pts',(-8.36880293377376,12.99372105772,49.7258548775597));
#19627=CARTESIAN_POINT('Ctrl Pts',(-14.7887116767695,12.8875648584764,48.2077926679319));
#19628=CARTESIAN_POINT('Ctrl Pts',(-26.6209452131421,12.6811033461879,42.8155264434361));
#19629=CARTESIAN_POINT('Ctrl Pts',(-31.9310851228465,12.5806516520033,39.0160191601527));
#19630=CARTESIAN_POINT('Ctrl Pts',(-40.8057542169951,12.3725378273868,29.6087010491045));
#19631=CARTESIAN_POINT('Ctrl Pts',(-44.2878907791481,12.2734177967731,24.0908202803128));
#19632=CARTESIAN_POINT('Ctrl Pts',(-48.9708157369014,12.0659484255844,12.0037061295532));
#19633=CARTESIAN_POINT('Ctrl Pts',(-50.1147724065617,11.9616918437045,5.54420998717902));
#19634=CARTESIAN_POINT('Ctrl Pts',(-49.8654311432801,11.7572567880282,-7.5357491602242));
#19635=CARTESIAN_POINT('Ctrl Pts',(-48.4409462355628,11.6503443297974,-14.0293652220786));
#19636=CARTESIAN_POINT('Ctrl Pts',(-43.1903182014914,11.4420551877761,-26.0170814558177));
#19637=CARTESIAN_POINT('Ctrl Pts',(-39.4439086950383,11.341475742409,-31.408120562985));
#19638=CARTESIAN_POINT('Ctrl Pts',(-30.1256355899705,11.1327501431137,-40.4255766808516));
#19639=CARTESIAN_POINT('Ctrl Pts',(-24.6527667112495,11.0334493868274,-43.9775217975006));
#19640=CARTESIAN_POINT('Ctrl Pts',(-12.6197365300443,10.8261700974901,-48.8166712331727));
#19641=CARTESIAN_POINT('Ctrl Pts',(-6.16767509119308,10.7210870421483,-50.0428165881525));
#19642=CARTESIAN_POINT('Ctrl Pts',(6.92971901291009,10.5170510432878,-49.9543171048813));
#19643=CARTESIAN_POINT('Ctrl Pts',(13.4481566577371,10.4100724633252,-48.6065983903204));
#19644=CARTESIAN_POINT('Ctrl Pts',(25.498360373273,10.2014016282185,-43.4975704726577));
#19645=CARTESIAN_POINT('Ctrl Pts',(30.9283498624805,10.1012198621366,-39.8201208804137));
#19646=CARTESIAN_POINT('Ctrl Pts',(40.0546020277859,9.89256933257104,-30.6172384055382));
#19647=CARTESIAN_POINT('Ctrl Pts',(43.6733473464145,9.79303668021819,-25.1878012179268));
#19648=CARTESIAN_POINT('Ctrl Pts',(48.6619829859239,9.58595245791768,-13.2073700775111));
#19649=CARTESIAN_POINT('Ctrl Pts',(49.9668720867691,9.4803009190459,-6.76279537354238));
#19650=CARTESIAN_POINT('Ctrl Pts',(50.0322701358121,9.27625560249255,6.34138794158945));
#19651=CARTESIAN_POINT('Ctrl Pts',(48.7616176208319,9.16964206396107,12.8742939124214));
#19652=CARTESIAN_POINT('Ctrl Pts',(43.7978146143124,8.96075145047578,24.9775439909932));
#19653=CARTESIAN_POINT('Ctrl Pts',(40.1891374783696,8.86091135354223,30.446006767238));
#19654=CARTESIAN_POINT('Ctrl Pts',(31.1014595076989,8.65234622350278,39.6799614216987));
#19655=CARTESIAN_POINT('Ctrl Pts',(25.7154264922144,8.55252643893411,43.3649295856025));
#19656=CARTESIAN_POINT('Ctrl Pts',(13.7882235291873,8.34565299031822,48.5016298032087));
#19657=CARTESIAN_POINT('Ctrl Pts',(7.35188535745777,8.23980419052421,49.884600682187));
#19658=CARTESIAN_POINT('Ctrl Pts',(0.55443206066175,8.13363112474586,49.9976954032747));
#19659=CARTESIAN_POINT('Ctrl Pts',(0.277164254761756,8.12930994918079,50.));
#19660=CARTESIAN_POINT('Ctrl Pts',(3.99680288865056E-14,8.12499998634407,
50.));
#19661=CARTESIAN_POINT('Ctrl Pts',(1.23512311489549E-14,8.75,50.));
#19662=CARTESIAN_POINT('Ctrl Pts',(0.648431293727216,8.7600832438892,50.));
#19663=CARTESIAN_POINT('Ctrl Pts',(1.29735475152641,8.77022669851377,49.9873862048369));
#19664=CARTESIAN_POINT('Ctrl Pts',(8.47721354847014,8.88304048381026,49.7076755550476));
#19665=CARTESIAN_POINT('Ctrl Pts',(14.8952044698391,8.98922696256952,48.1751888538927));
#19666=CARTESIAN_POINT('Ctrl Pts',(26.7170806653891,9.19564094423076,42.7556758577737));
#19667=CARTESIAN_POINT('Ctrl Pts',(32.0190546959999,9.29617028212578,38.9439377316323));
#19668=CARTESIAN_POINT('Ctrl Pts',(40.8728047658779,9.50427955327015,29.5161006010544));
#19669=CARTESIAN_POINT('Ctrl Pts',(44.3424804612446,9.60337391611804,23.9902255380222));
#19670=CARTESIAN_POINT('Ctrl Pts',(48.9975251595022,9.81087599828454,11.89353732302));
#19671=CARTESIAN_POINT('Ctrl Pts',(50.1268184516499,9.9149912031465,5.43274833024308));
#19672=CARTESIAN_POINT('Ctrl Pts',(49.8487676493035,10.119495407801,-7.64396493843533));
#19673=CARTESIAN_POINT('Ctrl Pts',(48.4106012754521,10.2263944461158,-14.1330520571305));
#19674=CARTESIAN_POINT('Ctrl Pts',(43.1347113770559,10.4346133937934,-26.1094853504774));
#19675=CARTESIAN_POINT('Ctrl Pts',(39.375966943307,10.5352697812222,-31.4935174489505));
#19676=CARTESIAN_POINT('Ctrl Pts',(30.0370674477733,10.7440076792621,-40.4914275730604));
#19677=CARTESIAN_POINT('Ctrl Pts',(24.5564395131693,10.8432729235818,-44.0313815757612));
#19678=CARTESIAN_POINT('Ctrl Pts',(12.5140651326065,11.0505856889662,-48.8436922359968));
#19679=CARTESIAN_POINT('Ctrl Pts',(6.06070339202204,11.1555226333687,-50.0557150028884));
#19680=CARTESIAN_POINT('Ctrl Pts',(-7.03378622739985,11.3596285829729,-49.9395876567563));
#19681=CARTESIAN_POINT('Ctrl Pts',(-13.5480267689982,11.4665968972053,-48.5786689149347));
#19682=CARTESIAN_POINT('Ctrl Pts',(-25.587584156021,11.6752035609711,-43.4453094801511));
#19683=CARTESIAN_POINT('Ctrl Pts',(-31.0109196299649,11.775449619827,-39.7560319739043));
#19684=CARTESIAN_POINT('Ctrl Pts',(-40.1185685393079,11.9841137816881,-30.5333486991097));
#19685=CARTESIAN_POINT('Ctrl Pts',(-43.7258848211684,12.0836026544728,-25.0964556960894));
#19686=CARTESIAN_POINT('Ctrl Pts',(-48.6889465030587,12.2907212194005,-13.1069635353675));
#19687=CARTESIAN_POINT('Ctrl Pts',(-49.9803639739704,12.3963372757602,-6.66106092154509));
#19688=CARTESIAN_POINT('Ctrl Pts',(-50.0194334783328,12.6002874467208,6.44405850153165));
#19689=CARTESIAN_POINT('Ctrl Pts',(-48.7348122369756,12.7070587862866,12.9764902577281));
#19690=CARTESIAN_POINT('Ctrl Pts',(-43.7439285895496,12.9159429418896,25.0720688081954));
#19691=CARTESIAN_POINT('Ctrl Pts',(-40.1228032384613,13.0158408141732,30.5335948218922));
#19692=CARTESIAN_POINT('Ctrl Pts',(-31.0142632226721,13.2244221739124,39.748113147005));
#19693=CARTESIAN_POINT('Ctrl Pts',(-25.6203671108846,13.3241858824379,43.4211235514659));
#19694=CARTESIAN_POINT('Ctrl Pts',(-13.6834613648333,13.5310988764741,48.5311033907353));
#19695=CARTESIAN_POINT('Ctrl Pts',(-7.24556749720559,13.6369131113857,49.8999727618044));
#19696=CARTESIAN_POINT('Ctrl Pts',(-0.484352129571248,13.742460893125,49.9982411063084));
#19697=CARTESIAN_POINT('Ctrl Pts',(-0.242136054053174,13.7462347330997,
50.));
#19698=CARTESIAN_POINT('Ctrl Pts',(-2.77555756156289E-16,13.75,50.));
#19699=CARTESIAN_POINT('Origin',(0.,30.,0.));
#19700=CARTESIAN_POINT('',(1.81713983480877E-14,18.75,50.));
#19701=CARTESIAN_POINT('',(-1.31924020975729E-14,18.1249999863441,50.));
#19702=CARTESIAN_POINT('',(-6.12323399573677E-15,30.,50.));
#19703=CARTESIAN_POINT('',(15.4508438171073,19.0004604433872,47.5528277323164));
#19704=CARTESIAN_POINT('Ctrl Pts',(1.66533453693773E-15,18.75,50.));
#19705=CARTESIAN_POINT('Ctrl Pts',(2.06343398963011,18.782086835364,50.));
#19706=CARTESIAN_POINT('Ctrl Pts',(4.12591617046045,18.8146910873865,49.8722678031709));
#19707=CARTESIAN_POINT('Ctrl Pts',(7.74823897426245,18.8728975253031,49.4214154483787));
#19708=CARTESIAN_POINT('Ctrl Pts',(9.31068297651482,18.8983205115452,49.1510191506797));
#19709=CARTESIAN_POINT('Ctrl Pts',(11.6326307868091,18.9365795554256,48.6344758199292));
#19710=CARTESIAN_POINT('Ctrl Pts',(12.4034070010999,18.9493604562429,48.4436356167657));
#19711=CARTESIAN_POINT('Ctrl Pts',(13.5522715319277,18.9685325039609,48.1299649645132));
#19712=CARTESIAN_POINT('Ctrl Pts',(13.9339731925082,18.9749226935498,48.020849453786));
#19713=CARTESIAN_POINT('Ctrl Pts',(14.5044722589624,18.9845043294477,47.8503883399713));
#19714=CARTESIAN_POINT('Ctrl Pts',(14.6942697542235,18.9876971505158,47.792445179082));
#19715=CARTESIAN_POINT('Ctrl Pts',(14.9784245353166,18.9924849931323,47.7038430313957));
#19716=CARTESIAN_POINT('Ctrl Pts',(15.0730437095848,18.9940805597343,47.6740306126352));
#19717=CARTESIAN_POINT('Ctrl Pts',(15.2148336244197,18.9964735029064,47.6288914175082));
#19718=CARTESIAN_POINT('Ctrl Pts',(15.2620713042067,18.9972710408533,47.6137757312423));
#19719=CARTESIAN_POINT('Ctrl Pts',(15.3610459806339,18.9989427577795,47.5819421900349));
#19720=CARTESIAN_POINT('Ctrl Pts',(15.4084466292325,18.9997437594921,47.5666034079044));
#19721=CARTESIAN_POINT('Ctrl Pts',(15.4508438170237,19.0004604433858,47.5528277323436));
#19722=CARTESIAN_POINT('',(15.450843269209,20.58,47.5528279103394));
#19723=CARTESIAN_POINT('',(15.4508436816103,19.3910854416803,47.5528277763422));
#19724=CARTESIAN_POINT('',(2.87173475049016,20.58,-49.9174632721138));
#19725=CARTESIAN_POINT('Origin',(0.,20.58,0.));
#19726=CARTESIAN_POINT('Ctrl Pts',(2.87173475049014,20.58,-49.9174632721138));
#19727=CARTESIAN_POINT('Ctrl Pts',(6.61637351959359,20.5208724585749,-49.7020354723747));
#19728=CARTESIAN_POINT('Ctrl Pts',(10.3248885349788,20.4605538158576,-49.0659276782243));
#19729=CARTESIAN_POINT('Ctrl Pts',(17.5213591482324,20.3399507406698,-46.978783597008));
#19730=CARTESIAN_POINT('Ctrl Pts',(20.9871203622869,20.2800466373442,-45.5361957365975));
#19731=CARTESIAN_POINT('Ctrl Pts',(29.9426187271194,20.1200818557983,-40.5670230702393));
#19732=CARTESIAN_POINT('Ctrl Pts',(34.9568796568864,20.0156924630395,-36.335402485389));
#19733=CARTESIAN_POINT('Ctrl Pts',(43.0625235284044,19.8082537643147,-26.2183663261997));
#19734=CARTESIAN_POINT('Ctrl Pts',(46.0878693059551,19.7091081425281,-20.4375102920327));
#19735=CARTESIAN_POINT('Ctrl Pts',(49.7830590432265,19.5003261545907,-8.00132178314007));
#19736=CARTESIAN_POINT('Ctrl Pts',(50.4008498182792,19.3993573063203,-1.45895842707427));
#19737=CARTESIAN_POINT('Ctrl Pts',(49.0875543111761,19.1914138579732,11.5615320758049));
#19738=CARTESIAN_POINT('Ctrl Pts',(47.1428011004522,19.0845709443303,17.9112704061328));
#19739=CARTESIAN_POINT('Ctrl Pts',(40.9471814385983,18.879806981529,29.419080354316));
#19740=CARTESIAN_POINT('Ctrl Pts',(36.7851237022354,18.7762175138932,34.4820162364731));
#19741=CARTESIAN_POINT('Ctrl Pts',(26.7798605317987,18.5685931862218,42.7157398751768));
#19742=CARTESIAN_POINT('Ctrl Pts',(21.0382551768946,18.4695789482211,45.8168863723286));
#19743=CARTESIAN_POINT('Ctrl Pts',(10.0448695016158,18.2843657945622,49.2401693631193));
#19744=CARTESIAN_POINT('Ctrl Pts',(5.03248290215808,18.2032561608402,50.));
#19745=CARTESIAN_POINT('Ctrl Pts',(-1.11022302462516E-14,18.1249999863441,
50.));
#19746=CARTESIAN_POINT('Origin',(0.,20.58,0.));
#19747=CARTESIAN_POINT('',(-6.4293956955236E-15,20.58,-52.5));
#19748=CARTESIAN_POINT('Origin',(0.,20.58,0.));
#19749=CARTESIAN_POINT('',(-6.4293956955236E-15,23.58,-52.5));
#19750=CARTESIAN_POINT('',(-6.4293956955236E-15,20.58,-52.5));
#19751=CARTESIAN_POINT('Origin',(0.,23.58,0.));
#19752=CARTESIAN_POINT('Origin',(0.,26.58,0.));
#19753=CARTESIAN_POINT('',(-6.4293956955236E-15,26.58,-52.5));
#19754=CARTESIAN_POINT('Origin',(0.,26.58,0.));
#19755=CARTESIAN_POINT('',(-6.4293956955236E-15,30.,-52.5));
#19756=CARTESIAN_POINT('',(-6.4293956955236E-15,26.58,-52.5));
#19757=CARTESIAN_POINT('Origin',(0.,30.,0.));
#19758=CARTESIAN_POINT('Origin',(0.,30.,0.));
#19759=CARTESIAN_POINT('',(-6.85802207522518E-15,0.,56.));
#19760=CARTESIAN_POINT('Origin',(0.,0.,0.));
#19761=CARTESIAN_POINT('',(-6.85802207522518E-15,30.,56.));
#19762=CARTESIAN_POINT('',(-6.85802207522518E-15,30.,56.));
#19763=CARTESIAN_POINT('Origin',(0.,30.,0.));
#19764=CARTESIAN_POINT('Origin',(0.,30.,0.));
#19765=CARTESIAN_POINT('',(-6.12323399573677E-15,26.58,50.));
#19766=CARTESIAN_POINT('Origin',(0.,26.58,0.));
#19767=CARTESIAN_POINT('',(-6.12323399573677E-15,23.58,50.));
#19768=CARTESIAN_POINT('',(-6.12323399573677E-15,30.,50.));
#19769=CARTESIAN_POINT('Origin',(0.,23.58,0.));
#19770=CARTESIAN_POINT('Origin',(0.,30.,0.));
#19771=CARTESIAN_POINT('Ctrl Pts',(0.,18.1249999863441,50.));
#19772=CARTESIAN_POINT('Ctrl Pts',(-1.46395213702768,18.1022352206972,50.));
#19773=CARTESIAN_POINT('Ctrl Pts',(-2.92959655005386,18.079176251773,49.9357068733922));
#19774=CARTESIAN_POINT('Ctrl Pts',(-10.9358446820847,17.9517352605888,49.2295937959252));
#19775=CARTESIAN_POINT('Ctrl Pts',(-17.3015950267471,17.8449930726363,47.3687724018939));
#19776=CARTESIAN_POINT('Ctrl Pts',(-28.8762103510446,17.6398472040909,41.3308164193438));
#19777=CARTESIAN_POINT('Ctrl Pts',(-33.9887542186337,17.5370136598723,37.2402609703136));
#19778=CARTESIAN_POINT('Ctrl Pts',(-42.3531696281848,17.3292115434088,27.3500715192646));
#19779=CARTESIAN_POINT('Ctrl Pts',(-45.5317450789481,17.2302636449031,21.6489612009597));
#19780=CARTESIAN_POINT('Ctrl Pts',(-49.5600708397194,17.0213776385416,9.29534702387663));
#19781=CARTESIAN_POINT('Ctrl Pts',(-50.3490242784998,16.9192661293503,2.75313777136309));
#19782=CARTESIAN_POINT('Ctrl Pts',(-49.3660254411158,16.7122378180411,-10.2970050021595));
#19783=CARTESIAN_POINT('Ctrl Pts',(-47.5907412654829,16.6056156676936,-16.677955620378));
#19784=CARTESIAN_POINT('Ctrl Pts',(-41.7136174652812,16.4001049116793,-28.3191309106804));
#19785=CARTESIAN_POINT('Ctrl Pts',(-37.6958122958252,16.2979713747829,-33.4817130582194));
#19786=CARTESIAN_POINT('Ctrl Pts',(-27.9228961236881,16.0900018004317,-41.9781122685046));
#19787=CARTESIAN_POINT('Ctrl Pts',(-22.2631451216861,15.9910509027763,-45.2349687866989));
#19788=CARTESIAN_POINT('Ctrl Pts',(-9.95302706610038,15.78213199501,-49.4335206200089));
#19789=CARTESIAN_POINT('Ctrl Pts',(-3.41151820394048,15.6793415211135,-50.3100090765765));
#19790=CARTESIAN_POINT('Ctrl Pts',(9.65163979754655,15.472811221036,-49.495106426816));
#19791=CARTESIAN_POINT('Ctrl Pts',(16.0467797762323,15.3663277979795,-47.8060722152372));
#19792=CARTESIAN_POINT('Ctrl Pts',(27.7535304462983,15.1604738188022,-42.0913055049256));
#19793=CARTESIAN_POINT('Ctrl Pts',(32.9660625462325,15.0589746911095,-38.1467601761831));
#19794=CARTESIAN_POINT('Ctrl Pts',(41.5943690684503,14.8508500890501,-28.49213273689));
#19795=CARTESIAN_POINT('Ctrl Pts',(44.929550902591,14.7518253890473,-22.874192221126));
#19796=CARTESIAN_POINT('Ctrl Pts',(49.2984439814791,14.5428875592743,-10.6085001319966));
#19797=CARTESIAN_POINT('Ctrl Pts',(50.2625783652768,14.4393542506304,-4.06812389386595));
#19798=CARTESIAN_POINT('Ctrl Pts',(49.6154032503147,14.2333425384376,9.00662731593866));
#19799=CARTESIAN_POINT('Ctrl Pts',(48.0124121338163,14.1270151373354,15.4147890428637));
#19800=CARTESIAN_POINT('Ctrl Pts',(42.459826826848,13.9208433441612,27.1854340099002));
#19801=CARTESIAN_POINT('Ctrl Pts',(38.5882949974709,13.8199061148943,32.4473144543822));
#19802=CARTESIAN_POINT('Ctrl Pts',(29.0517509449081,13.6116405034011,41.2060914917058));
#19803=CARTESIAN_POINT('Ctrl Pts',(23.4756436865131,13.5124727351935,44.6188352546216));
#19804=CARTESIAN_POINT('Ctrl Pts',(11.8301029936433,13.3133654493466,48.942834310463));
#19805=CARTESIAN_POINT('Ctrl Pts',(5.93604168035801,13.217306691123,50.));
#19806=CARTESIAN_POINT('Ctrl Pts',(-6.66133814775094E-15,13.1249999863441,
50.));
#19807=CARTESIAN_POINT('Ctrl Pts',(-2.66453525910038E-14,13.75,50.));
#19808=CARTESIAN_POINT('Ctrl Pts',(6.33436008535432,13.8485006402999,50.));
#19809=CARTESIAN_POINT('Ctrl Pts',(12.613801309995,13.9511629654864,48.796235648758));
#19810=CARTESIAN_POINT('Ctrl Pts',(24.5279767249908,14.1562049575921,44.0504655224356));
#19811=CARTESIAN_POINT('Ctrl Pts',(30.0291606250117,14.2557956626479,40.5007963959304));
#19812=CARTESIAN_POINT('Ctrl Pts',(39.3549009106075,14.464279263081,31.5120661140904));
#19813=CARTESIAN_POINT('Ctrl Pts',(43.0963799318702,14.5643893391982,26.1633465241914));
#19814=CARTESIAN_POINT('Ctrl Pts',(48.3592590130262,14.7710670457821,14.282540826403));
#19815=CARTESIAN_POINT('Ctrl Pts',(49.8088796826435,14.8770728815201,7.85396277520366));
#19816=CARTESIAN_POINT('Ctrl Pts',(50.1569070724122,15.08210598026,-5.2380123417253));
#19817=CARTESIAN_POINT('Ctrl Pts',(49.0356649182634,15.1871257413067,-11.7752530975039));
#19818=CARTESIAN_POINT('Ctrl Pts',(44.3616870702543,15.3960617215426,-23.9590790294512));
#19819=CARTESIAN_POINT('Ctrl Pts',(40.8862413681065,15.4953961484633,-29.5010488663333));
#19820=CARTESIAN_POINT('Ctrl Pts',(32.0221022500378,15.7037665326716,-38.9414347122342));
#19821=CARTESIAN_POINT('Ctrl Pts',(26.7204115323761,15.8042985976033,-42.7535968627668));
#19822=CARTESIAN_POINT('Ctrl Pts',(14.8988951547692,16.010710919205,-48.1740543034369));
#19823=CARTESIAN_POINT('Ctrl Pts',(8.48097128653307,16.1168984388664,-49.7070410668055));
#19824=CARTESIAN_POINT('Ctrl Pts',(-4.60218838353627,16.322472120921,-50.2177081476848));
#19825=CARTESIAN_POINT('Ctrl Pts',(-11.1413142841139,16.4266580876154,-49.1820099437241));
#19826=CARTESIAN_POINT('Ctrl Pts',(-23.3700742187699,16.6356008217794,-44.6741071340573));
#19827=CARTESIAN_POINT('Ctrl Pts',(-28.9535745488434,16.7347383572907,-41.2750124068013));
#19828=CARTESIAN_POINT('Ctrl Pts',(-38.5109673706576,16.9429800646524,-32.5391840233731));
#19829=CARTESIAN_POINT('Ctrl Pts',(-42.3953818478633,17.0440113346287,-27.2859794219456));
#19830=CARTESIAN_POINT('Ctrl Pts',(-47.976608376972,17.2501288144725,-15.5265016183736));
#19831=CARTESIAN_POINT('Ctrl Pts',(-49.5947857818058,17.3564850292136,-9.12055610322967));
#19832=CARTESIAN_POINT('Ctrl Pts',(-50.2715679782614,17.5625898545436,3.95224981457436));
#19833=CARTESIAN_POINT('Ctrl Pts',(-49.3229272811221,17.6659872998999,10.4928580226408));
#19834=CARTESIAN_POINT('Ctrl Pts',(-44.9841390385641,17.874922814359,22.7664677855985));
#19835=CARTESIAN_POINT('Ctrl Pts',(-41.6627992432918,17.9739293100305,28.3918287722335));
#19836=CARTESIAN_POINT('Ctrl Pts',(-33.0577929465509,18.1820274332102,38.0674303707594));
#19837=CARTESIAN_POINT('Ctrl Pts',(-27.8540797746203,18.2836338165375,42.0249568859643));
#19838=CARTESIAN_POINT('Ctrl Pts',(-16.158841993745,18.489428753646,47.7685201871846));
#19839=CARTESIAN_POINT('Ctrl Pts',(-9.76613431960756,18.5959380618995,49.4728443301955));
#19840=CARTESIAN_POINT('Ctrl Pts',(-2.15216982670219,18.7163885934413,49.9652695656877));
#19841=CARTESIAN_POINT('Ctrl Pts',(-1.07595777047503,18.7332686288908,50.));
#19842=CARTESIAN_POINT('Ctrl Pts',(2.77555756156289E-16,18.75,50.));
#19843=CARTESIAN_POINT('Origin',(15.2417684546534,19.3910854416803,46.909359659535));
#19844=CARTESIAN_POINT('',(15.2417680422519,20.58,46.9093597935322));
#19845=CARTESIAN_POINT('',(15.4508438171073,19.0004604433873,47.5528277323164));
#19846=CARTESIAN_POINT('Origin',(-4.44089209850063E-14,2.18749999317203,
-8.4502213867173E-14));
#19847=CARTESIAN_POINT('Ctrl Pts',(-47.293670625,5.31249999317204,-4.77048955893622E-15));
#19848=CARTESIAN_POINT('Ctrl Pts',(-47.293670625,5.52083332650537,12.6723008510722));
#19849=CARTESIAN_POINT('Ctrl Pts',(-40.9575201994638,5.7291666598387,23.6468353125));
#19850=CARTESIAN_POINT('Ctrl Pts',(-34.6213697739277,5.93749999317203,34.6213697739277));
#19851=CARTESIAN_POINT('Ctrl Pts',(-23.6468353125,6.14583332650537,40.9575201994638));
#19852=CARTESIAN_POINT('Ctrl Pts',(-12.6723008510723,6.3541666598387,47.293670625));
#19853=CARTESIAN_POINT('Ctrl Pts',(-2.77555756156289E-14,6.56249999317203,
47.293670625));
#19854=CARTESIAN_POINT('Ctrl Pts',(12.6723008510722,6.77083332650537,47.293670625));
#19855=CARTESIAN_POINT('Ctrl Pts',(23.6468353125,6.9791666598387,40.9575201994639));
#19856=CARTESIAN_POINT('Ctrl Pts',(34.6213697739277,7.18749999317204,34.6213697739278));
#19857=CARTESIAN_POINT('Ctrl Pts',(40.9575201994639,7.39583332650537,23.6468353125));
#19858=CARTESIAN_POINT('Ctrl Pts',(47.293670625,7.6041666598387,12.6723008510723));
#19859=CARTESIAN_POINT('Ctrl Pts',(47.293670625,7.81249999317203,4.33680868994202E-16));
#19860=CARTESIAN_POINT('Ctrl Pts',(47.293670625,8.02083332650537,-12.6723008510723));
#19861=CARTESIAN_POINT('Ctrl Pts',(40.9575201994639,8.2291666598387,-23.6468353125));
#19862=CARTESIAN_POINT('Ctrl Pts',(34.6213697739278,8.43749999317204,-34.6213697739277));
#19863=CARTESIAN_POINT('Ctrl Pts',(23.6468353125,8.64583332650537,-40.9575201994639));
#19864=CARTESIAN_POINT('Ctrl Pts',(12.6723008510723,8.8541666598387,-47.293670625));
#19865=CARTESIAN_POINT('Ctrl Pts',(0.,9.06249999317203,-47.293670625));
#19866=CARTESIAN_POINT('Ctrl Pts',(-12.6723008510723,9.27083332650536,-47.293670625));
#19867=CARTESIAN_POINT('Ctrl Pts',(-23.6468353125,9.4791666598387,-40.9575201994639));
#19868=CARTESIAN_POINT('Ctrl Pts',(-34.6213697739277,9.68749999317203,-34.6213697739277));
#19869=CARTESIAN_POINT('Ctrl Pts',(-40.9575201994638,9.89583332650537,-23.6468353125));
#19870=CARTESIAN_POINT('Ctrl Pts',(-47.293670625,10.1041666598387,-12.6723008510723));
#19871=CARTESIAN_POINT('Ctrl Pts',(-47.293670625,10.312499993172,-4.77048955893622E-15));
#19872=CARTESIAN_POINT('Ctrl Pts',(-47.293670625,4.06249999317204,-5.20417042793042E-15));
#19873=CARTESIAN_POINT('Ctrl Pts',(-47.293670625,4.27083332650536,12.6723008510722));
#19874=CARTESIAN_POINT('Ctrl Pts',(-40.9575201994638,4.4791666598387,23.6468353125));
#19875=CARTESIAN_POINT('Ctrl Pts',(-34.6213697739277,4.68749999317204,34.6213697739277));
#19876=CARTESIAN_POINT('Ctrl Pts',(-23.6468353125,4.89583332650537,40.9575201994639));
#19877=CARTESIAN_POINT('Ctrl Pts',(-12.6723008510723,5.1041666598387,47.293670625));
#19878=CARTESIAN_POINT('Ctrl Pts',(-2.77555756156289E-14,5.31249999317204,
47.293670625));
#19879=CARTESIAN_POINT('Ctrl Pts',(12.6723008510722,5.52083332650537,47.293670625));
#19880=CARTESIAN_POINT('Ctrl Pts',(23.6468353125,5.7291666598387,40.9575201994639));
#19881=CARTESIAN_POINT('Ctrl Pts',(34.6213697739277,5.93749999317203,34.6213697739278));
#19882=CARTESIAN_POINT('Ctrl Pts',(40.9575201994639,6.14583332650537,23.6468353125));
#19883=CARTESIAN_POINT('Ctrl Pts',(47.293670625,6.3541666598387,12.6723008510723));
#19884=CARTESIAN_POINT('Ctrl Pts',(47.293670625,6.56249999317203,0.));
#19885=CARTESIAN_POINT('Ctrl Pts',(47.293670625,6.77083332650537,-12.6723008510723));
#19886=CARTESIAN_POINT('Ctrl Pts',(40.9575201994639,6.9791666598387,-23.6468353125));
#19887=CARTESIAN_POINT('Ctrl Pts',(34.6213697739278,7.18749999317204,-34.6213697739277));
#19888=CARTESIAN_POINT('Ctrl Pts',(23.6468353125,7.39583332650537,-40.9575201994639));
#19889=CARTESIAN_POINT('Ctrl Pts',(12.6723008510723,7.6041666598387,-47.293670625));
#19890=CARTESIAN_POINT('Ctrl Pts',(0.,7.81249999317203,-47.293670625));
#19891=CARTESIAN_POINT('Ctrl Pts',(-12.6723008510723,8.02083332650537,-47.293670625));
#19892=CARTESIAN_POINT('Ctrl Pts',(-23.6468353125,8.2291666598387,-40.9575201994639));
#19893=CARTESIAN_POINT('Ctrl Pts',(-34.6213697739277,8.43749999317203,-34.6213697739278));
#19894=CARTESIAN_POINT('Ctrl Pts',(-40.9575201994638,8.64583332650537,-23.6468353125));
#19895=CARTESIAN_POINT('Ctrl Pts',(-47.293670625,8.8541666598387,-12.6723008510723));
#19896=CARTESIAN_POINT('Ctrl Pts',(-47.293670625,9.06249999317203,-5.20417042793042E-15));
#19897=CARTESIAN_POINT('Ctrl Pts',(50.,4.37499998634407,4.33680868994202E-16));
#19898=CARTESIAN_POINT('Ctrl Pts',(50.0000000000001,4.5833333196774,-13.3974596215561));
#19899=CARTESIAN_POINT('Ctrl Pts',(43.301270189222,4.79166665301074,-25.));
#19900=CARTESIAN_POINT('Ctrl Pts',(36.6025403784439,4.99999998634406,-36.6025403784439));
#19901=CARTESIAN_POINT('Ctrl Pts',(25.0000000000001,5.2083333196774,-43.3012701892219));
#19902=CARTESIAN_POINT('Ctrl Pts',(13.3974596215562,5.41666665301073,-50.));
#19903=CARTESIAN_POINT('Ctrl Pts',(2.77555756156289E-14,5.62499998634407,
-50.));
#19904=CARTESIAN_POINT('Ctrl Pts',(-13.3974596215561,5.8333333196774,-50.));
#19905=CARTESIAN_POINT('Ctrl Pts',(-25.,6.04166665301074,-43.301270189222));
#19906=CARTESIAN_POINT('Ctrl Pts',(-36.6025403784439,6.24999998634407,-36.6025403784439));
#19907=CARTESIAN_POINT('Ctrl Pts',(-43.3012701892219,6.4583333196774,-25.));
#19908=CARTESIAN_POINT('Ctrl Pts',(-50.,6.66666665301073,-13.3974596215561));
#19909=CARTESIAN_POINT('Ctrl Pts',(-50.,6.87499998634407,-5.63785129692462E-15));
#19910=CARTESIAN_POINT('Ctrl Pts',(-50.,7.0833333196774,13.3974596215561));
#19911=CARTESIAN_POINT('Ctrl Pts',(-43.3012701892219,7.29166665301073,25.));
#19912=CARTESIAN_POINT('Ctrl Pts',(-36.6025403784438,7.49999998634406,36.6025403784438));
#19913=CARTESIAN_POINT('Ctrl Pts',(-25.,7.7083333196774,43.3012701892219));
#19914=CARTESIAN_POINT('Ctrl Pts',(-13.3974596215562,7.91666665301074,50.));
#19915=CARTESIAN_POINT('Ctrl Pts',(0.,8.12499998634407,50.));
#19916=CARTESIAN_POINT('Ctrl Pts',(13.3974596215562,8.3333333196774,50.));
#19917=CARTESIAN_POINT('Ctrl Pts',(25.,8.54166665301073,43.301270189222));
#19918=CARTESIAN_POINT('Ctrl Pts',(36.6025403784438,8.74999998634407,36.6025403784439));
#19919=CARTESIAN_POINT('Ctrl Pts',(43.301270189222,8.9583333196774,25.));
#19920=CARTESIAN_POINT('Ctrl Pts',(50.,9.16666665301073,13.3974596215562));
#19921=CARTESIAN_POINT('Ctrl Pts',(50.,9.37499998634407,4.33680868994202E-16));
#19922=CARTESIAN_POINT('Ctrl Pts',(50.0000000000001,9.5833333196774,-13.3974596215561));
#19923=CARTESIAN_POINT('Ctrl Pts',(43.301270189222,9.79166665301073,-25.));
#19924=CARTESIAN_POINT('Ctrl Pts',(36.6025403784439,9.99999998634406,-36.6025403784439));
#19925=CARTESIAN_POINT('Ctrl Pts',(25.0000000000001,10.2083333196774,-43.3012701892219));
#19926=CARTESIAN_POINT('Ctrl Pts',(13.3974596215562,10.4166666530107,-50.));
#19927=CARTESIAN_POINT('Ctrl Pts',(2.77555756156289E-14,10.6249999863441,
-50.));
#19928=CARTESIAN_POINT('Ctrl Pts',(-13.3974596215561,10.8333333196774,-50.));
#19929=CARTESIAN_POINT('Ctrl Pts',(-25.,11.0416666530107,-43.301270189222));
#19930=CARTESIAN_POINT('Ctrl Pts',(-36.6025403784439,11.2499999863441,-36.6025403784439));
#19931=CARTESIAN_POINT('Ctrl Pts',(-43.3012701892219,11.4583333196774,-25.));
#19932=CARTESIAN_POINT('Ctrl Pts',(-50.,11.6666666530107,-13.3974596215561));
#19933=CARTESIAN_POINT('Ctrl Pts',(-50.,11.8749999863441,-5.63785129692462E-15));
#19934=CARTESIAN_POINT('Ctrl Pts',(-50.,12.0833333196774,13.3974596215561));
#19935=CARTESIAN_POINT('Ctrl Pts',(-43.3012701892219,12.2916666530107,25.));
#19936=CARTESIAN_POINT('Ctrl Pts',(-36.6025403784438,12.4999999863441,36.6025403784438));
#19937=CARTESIAN_POINT('Ctrl Pts',(-25.,12.7083333196774,43.3012701892219));
#19938=CARTESIAN_POINT('Ctrl Pts',(-13.3974596215562,12.9166666530107,50.));
#19939=CARTESIAN_POINT('Ctrl Pts',(0.,13.1249999863441,50.));
#19940=CARTESIAN_POINT('Ctrl Pts',(13.3974596215562,13.3333333196774,50.));
#19941=CARTESIAN_POINT('Ctrl Pts',(25.,13.5416666530107,43.301270189222));
#19942=CARTESIAN_POINT('Ctrl Pts',(36.6025403784438,13.7499999863441,36.6025403784439));
#19943=CARTESIAN_POINT('Ctrl Pts',(43.301270189222,13.9583333196774,25.));
#19944=CARTESIAN_POINT('Ctrl Pts',(50.,14.1666666530107,13.3974596215562));
#19945=CARTESIAN_POINT('Ctrl Pts',(50.,14.3749999863441,4.33680868994202E-16));
#19946=CARTESIAN_POINT('Ctrl Pts',(50.0000000000001,14.5833333196774,-13.3974596215561));
#19947=CARTESIAN_POINT('Ctrl Pts',(43.301270189222,14.7916666530107,-25.));
#19948=CARTESIAN_POINT('Ctrl Pts',(36.6025403784439,14.9999999863441,-36.6025403784439));
#19949=CARTESIAN_POINT('Ctrl Pts',(25.0000000000001,15.2083333196774,-43.3012701892219));
#19950=CARTESIAN_POINT('Ctrl Pts',(13.3974596215562,15.4166666530107,-50.));
#19951=CARTESIAN_POINT('Ctrl Pts',(2.77555756156289E-14,15.6249999863441,
-50.));
#19952=CARTESIAN_POINT('Ctrl Pts',(-13.3974596215561,15.8333333196774,-50.));
#19953=CARTESIAN_POINT('Ctrl Pts',(-25.,16.0416666530107,-43.301270189222));
#19954=CARTESIAN_POINT('Ctrl Pts',(-36.6025403784439,16.2499999863441,-36.6025403784439));
#19955=CARTESIAN_POINT('Ctrl Pts',(-43.3012701892219,16.4583333196774,-25.));
#19956=CARTESIAN_POINT('Ctrl Pts',(-50.,16.6666666530107,-13.3974596215561));
#19957=CARTESIAN_POINT('Ctrl Pts',(-50.,16.8749999863441,-5.63785129692462E-15));
#19958=CARTESIAN_POINT('Ctrl Pts',(-50.,17.0833333196774,13.3974596215561));
#19959=CARTESIAN_POINT('Ctrl Pts',(-43.3012701892219,17.2916666530107,25.));
#19960=CARTESIAN_POINT('Ctrl Pts',(-36.6025403784438,17.4999999863441,36.6025403784438));
#19961=CARTESIAN_POINT('Ctrl Pts',(-25.,17.7083333196774,43.3012701892219));
#19962=CARTESIAN_POINT('Ctrl Pts',(-13.3974596215562,17.9166666530107,50.));
#19963=CARTESIAN_POINT('Ctrl Pts',(0.,18.1249999863441,50.));
#19964=CARTESIAN_POINT('Ctrl Pts',(13.3974596215562,18.3333333196774,50.));
#19965=CARTESIAN_POINT('Ctrl Pts',(25.,18.5416666530107,43.301270189222));
#19966=CARTESIAN_POINT('Ctrl Pts',(36.6025403784438,18.7499999863441,36.6025403784439));
#19967=CARTESIAN_POINT('Ctrl Pts',(43.301270189222,18.9583333196774,25.));
#19968=CARTESIAN_POINT('Ctrl Pts',(50.,19.1666666530107,13.3974596215562));
#19969=CARTESIAN_POINT('Ctrl Pts',(50.,19.3749999863441,4.33680868994202E-16));
#19970=CARTESIAN_POINT('Ctrl Pts',(50.0000000000001,19.5833333196774,-13.3974596215561));
#19971=CARTESIAN_POINT('Ctrl Pts',(43.301270189222,19.7916666530107,-25.));
#19972=CARTESIAN_POINT('Ctrl Pts',(36.6025403784439,19.9999999863441,-36.6025403784439));
#19973=CARTESIAN_POINT('Ctrl Pts',(25.0000000000001,20.2083333196774,-43.3012701892219));
#19974=CARTESIAN_POINT('Ctrl Pts',(13.3974596215562,20.4166666530107,-50.));
#19975=CARTESIAN_POINT('Ctrl Pts',(2.77555756156289E-14,20.6249999863441,
-50.));
#19976=CARTESIAN_POINT('Ctrl Pts',(-13.3974596215561,20.8333333196774,-50.));
#19977=CARTESIAN_POINT('Ctrl Pts',(-25.,21.0416666530107,-43.301270189222));
#19978=CARTESIAN_POINT('Ctrl Pts',(-36.6025403784439,21.2499999863441,-36.6025403784439));
#19979=CARTESIAN_POINT('Ctrl Pts',(-43.3012701892219,21.4583333196774,-25.));
#19980=CARTESIAN_POINT('Ctrl Pts',(-50.,21.6666666530107,-13.3974596215561));
#19981=CARTESIAN_POINT('Ctrl Pts',(-50.,21.8749999863441,-5.63785129692462E-15));
#19982=CARTESIAN_POINT('Ctrl Pts',(-50.,22.0833333196774,13.3974596215561));
#19983=CARTESIAN_POINT('Ctrl Pts',(-43.3012701892219,22.2916666530107,25.));
#19984=CARTESIAN_POINT('Ctrl Pts',(-36.6025403784438,22.4999999863441,36.6025403784438));
#19985=CARTESIAN_POINT('Ctrl Pts',(-25.,22.7083333196774,43.3012701892219));
#19986=CARTESIAN_POINT('Ctrl Pts',(-13.3974596215562,22.9166666530107,50.));
#19987=CARTESIAN_POINT('Ctrl Pts',(0.,23.1249999863441,50.));
#19988=CARTESIAN_POINT('Ctrl Pts',(7.91921917061262,23.2481455209316,50.));
#19989=CARTESIAN_POINT('Ctrl Pts',(15.4508444385251,23.3754604402358,47.5528275304056));
#19990=CARTESIAN_POINT('Ctrl Pts',(47.293670625,2.81249999317203,4.33680868994202E-16));
#19991=CARTESIAN_POINT('Ctrl Pts',(47.293670625,3.02083332650537,-12.6723008510723));
#19992=CARTESIAN_POINT('Ctrl Pts',(40.9575201994639,3.2291666598387,-23.6468353125));
#19993=CARTESIAN_POINT('Ctrl Pts',(34.6213697739278,3.43749999317203,-34.6213697739277));
#19994=CARTESIAN_POINT('Ctrl Pts',(23.6468353125,3.64583332650537,-40.9575201994639));
#19995=CARTESIAN_POINT('Ctrl Pts',(12.6723008510723,3.8541666598387,-47.293670625));
#19996=CARTESIAN_POINT('Ctrl Pts',(0.,4.06249999317204,-47.293670625));
#19997=CARTESIAN_POINT('Ctrl Pts',(-12.6723008510723,4.27083332650536,-47.293670625));
#19998=CARTESIAN_POINT('Ctrl Pts',(-23.6468353125,4.4791666598387,-40.9575201994639));
#19999=CARTESIAN_POINT('Ctrl Pts',(-34.6213697739277,4.68749999317204,-34.6213697739277));
#20000=CARTESIAN_POINT('Ctrl Pts',(-40.9575201994638,4.89583332650537,-23.6468353125));
#20001=CARTESIAN_POINT('Ctrl Pts',(-47.293670625,5.1041666598387,-12.6723008510723));
#20002=CARTESIAN_POINT('Ctrl Pts',(-47.293670625,5.31249999317204,-4.77048955893622E-15));
#20003=CARTESIAN_POINT('Ctrl Pts',(-47.293670625,5.52083332650537,12.6723008510722));
#20004=CARTESIAN_POINT('Ctrl Pts',(-40.9575201994638,5.7291666598387,23.6468353125));
#20005=CARTESIAN_POINT('Ctrl Pts',(-34.6213697739277,5.93749999317203,34.6213697739277));
#20006=CARTESIAN_POINT('Ctrl Pts',(-23.6468353125,6.14583332650537,40.9575201994638));
#20007=CARTESIAN_POINT('Ctrl Pts',(-12.6723008510723,6.3541666598387,47.293670625));
#20008=CARTESIAN_POINT('Ctrl Pts',(-2.77555756156289E-14,6.56249999317203,
47.293670625));
#20009=CARTESIAN_POINT('Ctrl Pts',(12.6723008510722,6.77083332650537,47.293670625));
#20010=CARTESIAN_POINT('Ctrl Pts',(23.6468353125,6.9791666598387,40.9575201994639));
#20011=CARTESIAN_POINT('Ctrl Pts',(34.6213697739277,7.18749999317204,34.6213697739278));
#20012=CARTESIAN_POINT('Ctrl Pts',(40.9575201994639,7.39583332650537,23.6468353125));
#20013=CARTESIAN_POINT('Ctrl Pts',(47.293670625,7.6041666598387,12.6723008510723));
#20014=CARTESIAN_POINT('Ctrl Pts',(47.293670625,7.81249999317203,4.33680868994202E-16));
#20015=CARTESIAN_POINT('Ctrl Pts',(47.293670625,8.02083332650537,-12.6723008510723));
#20016=CARTESIAN_POINT('Ctrl Pts',(40.9575201994639,8.2291666598387,-23.6468353125));
#20017=CARTESIAN_POINT('Ctrl Pts',(34.6213697739278,8.43749999317204,-34.6213697739277));
#20018=CARTESIAN_POINT('Ctrl Pts',(23.6468353125,8.64583332650537,-40.9575201994639));
#20019=CARTESIAN_POINT('Ctrl Pts',(12.6723008510723,8.8541666598387,-47.293670625));
#20020=CARTESIAN_POINT('Ctrl Pts',(0.,9.06249999317203,-47.293670625));
#20021=CARTESIAN_POINT('Ctrl Pts',(-12.6723008510723,9.27083332650537,-47.293670625));
#20022=CARTESIAN_POINT('Ctrl Pts',(-23.6468353125,9.4791666598387,-40.9575201994639));
#20023=CARTESIAN_POINT('Ctrl Pts',(-34.6213697739277,9.68749999317203,-34.6213697739277));
#20024=CARTESIAN_POINT('Ctrl Pts',(-40.9575201994638,9.89583332650537,-23.6468353125));
#20025=CARTESIAN_POINT('Ctrl Pts',(-47.293670625,10.1041666598387,-12.6723008510723));
#20026=CARTESIAN_POINT('Ctrl Pts',(-47.293670625,10.312499993172,-4.77048955893622E-15));
#20027=CARTESIAN_POINT('Ctrl Pts',(-47.293670625,10.5208333265054,12.6723008510722));
#20028=CARTESIAN_POINT('Ctrl Pts',(-40.9575201994638,10.7291666598387,23.6468353125));
#20029=CARTESIAN_POINT('Ctrl Pts',(-34.6213697739277,10.937499993172,34.6213697739277));
#20030=CARTESIAN_POINT('Ctrl Pts',(-23.6468353125,11.1458333265054,40.9575201994638));
#20031=CARTESIAN_POINT('Ctrl Pts',(-12.6723008510723,11.3541666598387,47.293670625));
#20032=CARTESIAN_POINT('Ctrl Pts',(-2.77555756156289E-14,11.562499993172,
47.293670625));
#20033=CARTESIAN_POINT('Ctrl Pts',(12.6723008510722,11.7708333265054,47.293670625));
#20034=CARTESIAN_POINT('Ctrl Pts',(23.6468353125,11.9791666598387,40.9575201994639));
#20035=CARTESIAN_POINT('Ctrl Pts',(34.6213697739277,12.187499993172,34.6213697739278));
#20036=CARTESIAN_POINT('Ctrl Pts',(40.9575201994639,12.3958333265054,23.6468353125));
#20037=CARTESIAN_POINT('Ctrl Pts',(47.293670625,12.6041666598387,12.6723008510723));
#20038=CARTESIAN_POINT('Ctrl Pts',(47.293670625,12.812499993172,4.33680868994202E-16));
#20039=CARTESIAN_POINT('Ctrl Pts',(47.293670625,13.0208333265054,-12.6723008510723));
#20040=CARTESIAN_POINT('Ctrl Pts',(40.9575201994639,13.2291666598387,-23.6468353125));
#20041=CARTESIAN_POINT('Ctrl Pts',(34.6213697739278,13.437499993172,-34.6213697739277));
#20042=CARTESIAN_POINT('Ctrl Pts',(23.6468353125,13.6458333265054,-40.9575201994639));
#20043=CARTESIAN_POINT('Ctrl Pts',(12.6723008510723,13.8541666598387,-47.293670625));
#20044=CARTESIAN_POINT('Ctrl Pts',(0.,14.062499993172,-47.293670625));
#20045=CARTESIAN_POINT('Ctrl Pts',(-12.6723008510723,14.2708333265054,-47.293670625));
#20046=CARTESIAN_POINT('Ctrl Pts',(-23.6468353125,14.4791666598387,-40.9575201994639));
#20047=CARTESIAN_POINT('Ctrl Pts',(-34.6213697739277,14.687499993172,-34.6213697739277));
#20048=CARTESIAN_POINT('Ctrl Pts',(-40.9575201994638,14.8958333265054,-23.6468353125));
#20049=CARTESIAN_POINT('Ctrl Pts',(-47.293670625,15.1041666598387,-12.6723008510723));
#20050=CARTESIAN_POINT('Ctrl Pts',(-47.293670625,15.312499993172,-4.77048955893622E-15));
#20051=CARTESIAN_POINT('Ctrl Pts',(-47.293670625,15.5208333265054,12.6723008510722));
#20052=CARTESIAN_POINT('Ctrl Pts',(-40.9575201994638,15.7291666598387,23.6468353125));
#20053=CARTESIAN_POINT('Ctrl Pts',(-34.6213697739277,15.937499993172,34.6213697739277));
#20054=CARTESIAN_POINT('Ctrl Pts',(-23.6468353125,16.1458333265054,40.9575201994638));
#20055=CARTESIAN_POINT('Ctrl Pts',(-12.6723008510723,16.3541666598387,47.293670625));
#20056=CARTESIAN_POINT('Ctrl Pts',(-2.77555756156289E-14,16.562499993172,
47.293670625));
#20057=CARTESIAN_POINT('Ctrl Pts',(12.6723008510722,16.7708333265054,47.293670625));
#20058=CARTESIAN_POINT('Ctrl Pts',(23.6468353125,16.9791666598387,40.9575201994639));
#20059=CARTESIAN_POINT('Ctrl Pts',(34.6213697739277,17.187499993172,34.6213697739278));
#20060=CARTESIAN_POINT('Ctrl Pts',(40.9575201994639,17.3958333265054,23.6468353125));
#20061=CARTESIAN_POINT('Ctrl Pts',(47.293670625,17.6041666598387,12.6723008510723));
#20062=CARTESIAN_POINT('Ctrl Pts',(47.293670625,17.812499993172,4.33680868994202E-16));
#20063=CARTESIAN_POINT('Ctrl Pts',(47.293670625,18.0208333265054,-12.6723008510723));
#20064=CARTESIAN_POINT('Ctrl Pts',(40.9575201994639,18.2291666598387,-23.6468353125));
#20065=CARTESIAN_POINT('Ctrl Pts',(34.6213697739278,18.437499993172,-34.6213697739277));
#20066=CARTESIAN_POINT('Ctrl Pts',(23.6468353125,18.6458333265054,-40.9575201994639));
#20067=CARTESIAN_POINT('Ctrl Pts',(12.6723008510723,18.8541666598387,-47.293670625));
#20068=CARTESIAN_POINT('Ctrl Pts',(0.,19.062499993172,-47.293670625));
#20069=CARTESIAN_POINT('Ctrl Pts',(-12.6723008510723,19.2708333265054,-47.293670625));
#20070=CARTESIAN_POINT('Ctrl Pts',(-23.6468353125,19.4791666598387,-40.9575201994639));
#20071=CARTESIAN_POINT('Ctrl Pts',(-34.6213697739277,19.687499993172,-34.6213697739277));
#20072=CARTESIAN_POINT('Ctrl Pts',(-40.9575201994638,19.8958333265054,-23.6468353125));
#20073=CARTESIAN_POINT('Ctrl Pts',(-47.293670625,20.1041666598387,-12.6723008510723));
#20074=CARTESIAN_POINT('Ctrl Pts',(-47.293670625,20.312499993172,-4.77048955893622E-15));
#20075=CARTESIAN_POINT('Ctrl Pts',(-47.293670625,20.5208333265054,12.6723008510722));
#20076=CARTESIAN_POINT('Ctrl Pts',(-40.9575201994638,20.7291666598387,23.6468353125));
#20077=CARTESIAN_POINT('Ctrl Pts',(-34.6213697739277,20.937499993172,34.6213697739277));
#20078=CARTESIAN_POINT('Ctrl Pts',(-23.6468353125,21.1458333265054,40.9575201994638));
#20079=CARTESIAN_POINT('Ctrl Pts',(-12.6723008510723,21.3541666598387,47.293670625));
#20080=CARTESIAN_POINT('Ctrl Pts',(-2.77555756156289E-14,21.562499993172,
47.293670625));
#20081=CARTESIAN_POINT('Ctrl Pts',(7.49057886124279,21.6856455277595,47.293670625));
#20082=CARTESIAN_POINT('Ctrl Pts',(14.6145429550743,21.8129604470638,44.9789552502087));
#20083=CARTESIAN_POINT('Ctrl Pts',(-44.6588684919844,20.58,15.5652416043447));
#20084=CARTESIAN_POINT('Ctrl Pts',(-45.8223695666528,20.58,12.5182222321844));
#20085=CARTESIAN_POINT('Ctrl Pts',(-46.6680986770167,20.58,9.35920006449212));
#20086=CARTESIAN_POINT('Ctrl Pts',(-47.7115459842877,20.58,2.82738845179393));
#20087=CARTESIAN_POINT('Ctrl Pts',(-47.8846290450767,20.58,-0.526241684364264));
#20088=CARTESIAN_POINT('Ctrl Pts',(-47.3912185290812,20.58,-9.99324512899516));
#20089=CARTESIAN_POINT('Ctrl Pts',(-45.8995255488925,20.58,-16.0093794384006));
#20090=CARTESIAN_POINT('Ctrl Pts',(-41.9677631661302,20.58,-24.4923235135627));
#20091=CARTESIAN_POINT('Ctrl Pts',(-40.327232006205,20.58,-27.2658254068393));
#20092=CARTESIAN_POINT('Ctrl Pts',(-36.5713996983444,20.58,-32.3974946095854));
#20093=CARTESIAN_POINT('Ctrl Pts',(-34.4608877029428,20.58,-34.761199114609));
#20094=CARTESIAN_POINT('Ctrl Pts',(-27.0961825388857,20.58,-41.551889627277));
#20095=CARTESIAN_POINT('Ctrl Pts',(-21.4281170361254,20.5799999999902,-44.8194014831955));
#20096=CARTESIAN_POINT('Ctrl Pts',(-12.7851969301205,20.5799999999902,-47.9873865019175));
#20097=CARTESIAN_POINT('Ctrl Pts',(-9.76123390768821,20.58,-48.7819503108552));
#20098=CARTESIAN_POINT('Ctrl Pts',(-3.52062841150329,20.58,-49.8054784288519));
#20099=CARTESIAN_POINT('Ctrl Pts',(-0.322512932949123,20.58,-50.0138607547272));
#20100=CARTESIAN_POINT('Ctrl Pts',(2.87173475049018,20.58,-49.9174632721138));
#20101=CARTESIAN_POINT('',(50.,4.37499998634407,4.33680868994202E-16));
#20102=CARTESIAN_POINT('Origin',(0.,30.,0.));
#20103=CARTESIAN_POINT('Origin',(0.,0.,0.));
#20104=CARTESIAN_POINT('Origin',(48.6468353125001,0.78124999658602,4.33680868994202E-16));
#20105=CARTESIAN_POINT('',(47.293670625,1.56249999317203,0.));
#20106=CARTESIAN_POINT('Ctrl Pts',(47.293670625,1.56249999317203,0.));
#20107=CARTESIAN_POINT('Ctrl Pts',(47.293670625,1.77083332650536,-12.6723008510723));
#20108=CARTESIAN_POINT('Ctrl Pts',(40.9575201994639,1.9791666598387,-23.6468353125));
#20109=CARTESIAN_POINT('Ctrl Pts',(34.6213697739278,2.18749999317203,-34.6213697739277));
#20110=CARTESIAN_POINT('Ctrl Pts',(23.6468353125,2.39583332650536,-40.9575201994639));
#20111=CARTESIAN_POINT('Ctrl Pts',(12.6723008510723,2.6041666598387,-47.293670625));
#20112=CARTESIAN_POINT('Ctrl Pts',(0.,2.81249999317203,-47.293670625));
#20113=CARTESIAN_POINT('Ctrl Pts',(-12.6723008510723,3.02083332650537,-47.293670625));
#20114=CARTESIAN_POINT('Ctrl Pts',(-23.6468353125,3.2291666598387,-40.9575201994639));
#20115=CARTESIAN_POINT('Ctrl Pts',(-34.6213697739277,3.43749999317203,-34.6213697739278));
#20116=CARTESIAN_POINT('Ctrl Pts',(-40.9575201994638,3.64583332650537,-23.6468353125));
#20117=CARTESIAN_POINT('Ctrl Pts',(-47.293670625,3.8541666598387,-12.6723008510723));
#20118=CARTESIAN_POINT('Ctrl Pts',(-47.293670625,4.06249999317204,-5.20417042793042E-15));
#20119=CARTESIAN_POINT('Ctrl Pts',(-47.293670625,4.27083332650536,12.6723008510722));
#20120=CARTESIAN_POINT('Ctrl Pts',(-40.9575201994638,4.4791666598387,23.6468353125));
#20121=CARTESIAN_POINT('Ctrl Pts',(-34.6213697739277,4.68749999317204,34.6213697739277));
#20122=CARTESIAN_POINT('Ctrl Pts',(-23.6468353125,4.89583332650537,40.9575201994639));
#20123=CARTESIAN_POINT('Ctrl Pts',(-12.6723008510723,5.1041666598387,47.293670625));
#20124=CARTESIAN_POINT('Ctrl Pts',(-2.77555756156289E-14,5.31249999317204,
47.293670625));
#20125=CARTESIAN_POINT('Ctrl Pts',(12.6723008510722,5.52083332650537,47.293670625));
#20126=CARTESIAN_POINT('Ctrl Pts',(23.6468353125,5.7291666598387,40.9575201994639));
#20127=CARTESIAN_POINT('Ctrl Pts',(34.6213697739277,5.93749999317203,34.6213697739278));
#20128=CARTESIAN_POINT('Ctrl Pts',(40.9575201994639,6.14583332650537,23.6468353125));
#20129=CARTESIAN_POINT('Ctrl Pts',(47.293670625,6.3541666598387,12.6723008510723));
#20130=CARTESIAN_POINT('Ctrl Pts',(47.293670625,6.56249999317203,0.));
#20131=CARTESIAN_POINT('Ctrl Pts',(47.293670625,6.77083332650537,-12.6723008510723));
#20132=CARTESIAN_POINT('Ctrl Pts',(40.9575201994639,6.9791666598387,-23.6468353125));
#20133=CARTESIAN_POINT('Ctrl Pts',(34.6213697739278,7.18749999317204,-34.6213697739277));
#20134=CARTESIAN_POINT('Ctrl Pts',(23.6468353125,7.39583332650537,-40.9575201994639));
#20135=CARTESIAN_POINT('Ctrl Pts',(12.6723008510723,7.6041666598387,-47.293670625));
#20136=CARTESIAN_POINT('Ctrl Pts',(0.,7.81249999317203,-47.293670625));
#20137=CARTESIAN_POINT('Ctrl Pts',(-12.6723008510723,8.02083332650537,-47.293670625));
#20138=CARTESIAN_POINT('Ctrl Pts',(-23.6468353125,8.2291666598387,-40.9575201994639));
#20139=CARTESIAN_POINT('Ctrl Pts',(-34.6213697739277,8.43749999317203,-34.6213697739278));
#20140=CARTESIAN_POINT('Ctrl Pts',(-40.9575201994638,8.64583332650537,-23.6468353125));
#20141=CARTESIAN_POINT('Ctrl Pts',(-47.293670625,8.8541666598387,-12.6723008510723));
#20142=CARTESIAN_POINT('Ctrl Pts',(-47.293670625,9.06249999317203,-5.20417042793042E-15));
#20143=CARTESIAN_POINT('Ctrl Pts',(-47.293670625,9.27083332650537,12.6723008510722));
#20144=CARTESIAN_POINT('Ctrl Pts',(-40.9575201994638,9.4791666598387,23.6468353125));
#20145=CARTESIAN_POINT('Ctrl Pts',(-34.6213697739277,9.68749999317203,34.6213697739277));
#20146=CARTESIAN_POINT('Ctrl Pts',(-23.6468353125,9.89583332650536,40.9575201994639));
#20147=CARTESIAN_POINT('Ctrl Pts',(-12.6723008510723,10.1041666598387,47.293670625));
#20148=CARTESIAN_POINT('Ctrl Pts',(-2.77555756156289E-14,10.312499993172,
47.293670625));
#20149=CARTESIAN_POINT('Ctrl Pts',(12.6723008510722,10.5208333265054,47.293670625));
#20150=CARTESIAN_POINT('Ctrl Pts',(23.6468353125,10.7291666598387,40.9575201994639));
#20151=CARTESIAN_POINT('Ctrl Pts',(34.6213697739277,10.937499993172,34.6213697739278));
#20152=CARTESIAN_POINT('Ctrl Pts',(40.9575201994639,11.1458333265054,23.6468353125));
#20153=CARTESIAN_POINT('Ctrl Pts',(47.293670625,11.3541666598387,12.6723008510723));
#20154=CARTESIAN_POINT('Ctrl Pts',(47.293670625,11.562499993172,0.));
#20155=CARTESIAN_POINT('Ctrl Pts',(47.293670625,11.7708333265054,-12.6723008510723));
#20156=CARTESIAN_POINT('Ctrl Pts',(40.9575201994639,11.9791666598387,-23.6468353125));
#20157=CARTESIAN_POINT('Ctrl Pts',(34.6213697739278,12.187499993172,-34.6213697739277));
#20158=CARTESIAN_POINT('Ctrl Pts',(23.6468353125,12.3958333265054,-40.9575201994639));
#20159=CARTESIAN_POINT('Ctrl Pts',(12.6723008510723,12.6041666598387,-47.293670625));
#20160=CARTESIAN_POINT('Ctrl Pts',(0.,12.812499993172,-47.293670625));
#20161=CARTESIAN_POINT('Ctrl Pts',(-12.6723008510723,13.0208333265054,-47.293670625));
#20162=CARTESIAN_POINT('Ctrl Pts',(-23.6468353125,13.2291666598387,-40.9575201994639));
#20163=CARTESIAN_POINT('Ctrl Pts',(-34.6213697739277,13.437499993172,-34.6213697739278));
#20164=CARTESIAN_POINT('Ctrl Pts',(-40.9575201994638,13.6458333265054,-23.6468353125));
#20165=CARTESIAN_POINT('Ctrl Pts',(-47.293670625,13.8541666598387,-12.6723008510723));
#20166=CARTESIAN_POINT('Ctrl Pts',(-47.293670625,14.062499993172,-5.20417042793042E-15));
#20167=CARTESIAN_POINT('Ctrl Pts',(-47.293670625,14.2708333265054,12.6723008510722));
#20168=CARTESIAN_POINT('Ctrl Pts',(-40.9575201994638,14.4791666598387,23.6468353125));
#20169=CARTESIAN_POINT('Ctrl Pts',(-34.6213697739277,14.687499993172,34.6213697739277));
#20170=CARTESIAN_POINT('Ctrl Pts',(-23.6468353125,14.8958333265054,40.9575201994639));
#20171=CARTESIAN_POINT('Ctrl Pts',(-12.6723008510723,15.1041666598387,47.293670625));
#20172=CARTESIAN_POINT('Ctrl Pts',(-2.77555756156289E-14,15.312499993172,
47.293670625));
#20173=CARTESIAN_POINT('Ctrl Pts',(12.6723008510722,15.5208333265054,47.293670625));
#20174=CARTESIAN_POINT('Ctrl Pts',(23.6468353125,15.7291666598387,40.9575201994639));
#20175=CARTESIAN_POINT('Ctrl Pts',(34.6213697739277,15.937499993172,34.6213697739278));
#20176=CARTESIAN_POINT('Ctrl Pts',(40.9575201994639,16.1458333265054,23.6468353125));
#20177=CARTESIAN_POINT('Ctrl Pts',(47.293670625,16.3541666598387,12.6723008510723));
#20178=CARTESIAN_POINT('Ctrl Pts',(47.293670625,16.562499993172,0.));
#20179=CARTESIAN_POINT('Ctrl Pts',(47.293670625,16.7708333265054,-12.6723008510723));
#20180=CARTESIAN_POINT('Ctrl Pts',(40.9575201994639,16.9791666598387,-23.6468353125));
#20181=CARTESIAN_POINT('Ctrl Pts',(34.6213697739278,17.187499993172,-34.6213697739277));
#20182=CARTESIAN_POINT('Ctrl Pts',(23.6468353125,17.3958333265054,-40.9575201994639));
#20183=CARTESIAN_POINT('Ctrl Pts',(12.6723008510723,17.6041666598387,-47.293670625));
#20184=CARTESIAN_POINT('Ctrl Pts',(0.,17.812499993172,-47.293670625));
#20185=CARTESIAN_POINT('Ctrl Pts',(-12.6723008510723,18.0208333265054,-47.293670625));
#20186=CARTESIAN_POINT('Ctrl Pts',(-23.6468353125,18.2291666598387,-40.9575201994639));
#20187=CARTESIAN_POINT('Ctrl Pts',(-34.6213697739277,18.437499993172,-34.6213697739278));
#20188=CARTESIAN_POINT('Ctrl Pts',(-40.9575201994638,18.6458333265054,-23.6468353125));
#20189=CARTESIAN_POINT('Ctrl Pts',(-47.293670625,18.8541666598387,-12.6723008510723));
#20190=CARTESIAN_POINT('Ctrl Pts',(-47.293670625,19.062499993172,-5.20417042793042E-15));
#20191=CARTESIAN_POINT('Ctrl Pts',(-47.293670625,19.2708333265054,12.6723008510722));
#20192=CARTESIAN_POINT('Ctrl Pts',(-40.9575201994638,19.4791666598387,23.6468353125));
#20193=CARTESIAN_POINT('Ctrl Pts',(-34.6213697739277,19.687499993172,34.6213697739277));
#20194=CARTESIAN_POINT('Ctrl Pts',(-23.6468353125,19.8958333265054,40.9575201994639));
#20195=CARTESIAN_POINT('Ctrl Pts',(-12.6723008510723,20.1041666598387,47.293670625));
#20196=CARTESIAN_POINT('Ctrl Pts',(-2.77555756156289E-14,20.312499993172,
47.293670625));
#20197=CARTESIAN_POINT('Ctrl Pts',(7.49057854447537,20.4356455225519,47.293670625));
#20198=CARTESIAN_POINT('Ctrl Pts',(14.6145423672918,20.5629604365593,44.9789554411907));
#20199=CARTESIAN_POINT('Ctrl Pts',(20.0112685210152,20.65940726634,43.2254535591521));
#20200=CARTESIAN_POINT('Ctrl Pts',(25.4079946747386,20.7558540961206,41.4719516771133));
#20201=CARTESIAN_POINT('Ctrl Pts',(50.,0.,4.33680868994202E-16));
#20202=CARTESIAN_POINT('Ctrl Pts',(50.0000000000001,0.208333333333332,-13.3974596215561));
#20203=CARTESIAN_POINT('Ctrl Pts',(43.301270189222,0.416666666666669,-25.));
#20204=CARTESIAN_POINT('Ctrl Pts',(36.6025403784439,0.625000000000002,-36.6025403784439));
#20205=CARTESIAN_POINT('Ctrl Pts',(25.0000000000001,0.833333333333332,-43.3012701892219));
#20206=CARTESIAN_POINT('Ctrl Pts',(13.3974596215562,1.04166666666667,-50.));
#20207=CARTESIAN_POINT('Ctrl Pts',(2.77555756156289E-14,1.25,-50.));
#20208=CARTESIAN_POINT('Ctrl Pts',(-13.3974596215561,1.45833333333334,-50.));
#20209=CARTESIAN_POINT('Ctrl Pts',(-25.,1.66666666666666,-43.301270189222));
#20210=CARTESIAN_POINT('Ctrl Pts',(-36.6025403784439,1.875,-36.6025403784439));
#20211=CARTESIAN_POINT('Ctrl Pts',(-43.3012701892219,2.08333333333333,-25.));
#20212=CARTESIAN_POINT('Ctrl Pts',(-50.,2.29166666666667,-13.3974596215561));
#20213=CARTESIAN_POINT('Ctrl Pts',(-50.,2.5,-5.63785129692462E-15));
#20214=CARTESIAN_POINT('Ctrl Pts',(-50.,2.70833333333333,13.3974596215561));
#20215=CARTESIAN_POINT('Ctrl Pts',(-43.3012701892219,2.91666666666666,25.));
#20216=CARTESIAN_POINT('Ctrl Pts',(-36.6025403784438,3.125,36.6025403784438));
#20217=CARTESIAN_POINT('Ctrl Pts',(-25.,3.33333333333333,43.3012701892219));
#20218=CARTESIAN_POINT('Ctrl Pts',(-13.3974596215562,3.54166666666667,50.));
#20219=CARTESIAN_POINT('Ctrl Pts',(0.,3.75,50.));
#20220=CARTESIAN_POINT('Ctrl Pts',(13.3974596215562,3.95833333333334,50.));
#20221=CARTESIAN_POINT('Ctrl Pts',(25.,4.16666666666667,43.301270189222));
#20222=CARTESIAN_POINT('Ctrl Pts',(36.6025403784438,4.375,36.6025403784439));
#20223=CARTESIAN_POINT('Ctrl Pts',(43.301270189222,4.58333333333333,25.));
#20224=CARTESIAN_POINT('Ctrl Pts',(50.,4.79166666666667,13.3974596215562));
#20225=CARTESIAN_POINT('Ctrl Pts',(50.,5.,4.33680868994202E-16));
#20226=CARTESIAN_POINT('Ctrl Pts',(50.0000000000001,5.20833333333333,-13.3974596215561));
#20227=CARTESIAN_POINT('Ctrl Pts',(43.301270189222,5.41666666666667,-25.));
#20228=CARTESIAN_POINT('Ctrl Pts',(36.6025403784439,5.62499999999999,-36.6025403784439));
#20229=CARTESIAN_POINT('Ctrl Pts',(25.0000000000001,5.83333333333333,-43.3012701892219));
#20230=CARTESIAN_POINT('Ctrl Pts',(13.3974596215562,6.04166666666667,-50.));
#20231=CARTESIAN_POINT('Ctrl Pts',(2.77555756156289E-14,6.25,-50.));
#20232=CARTESIAN_POINT('Ctrl Pts',(-13.3974596215561,6.45833333333334,-50.));
#20233=CARTESIAN_POINT('Ctrl Pts',(-25.,6.66666666666667,-43.301270189222));
#20234=CARTESIAN_POINT('Ctrl Pts',(-36.6025403784439,6.875,-36.6025403784439));
#20235=CARTESIAN_POINT('Ctrl Pts',(-43.3012701892219,7.08333333333333,-25.));
#20236=CARTESIAN_POINT('Ctrl Pts',(-50.,7.29166666666666,-13.3974596215561));
#20237=CARTESIAN_POINT('Ctrl Pts',(-50.,7.5,-5.63785129692462E-15));
#20238=CARTESIAN_POINT('Ctrl Pts',(-50.,7.70833333333333,13.3974596215561));
#20239=CARTESIAN_POINT('Ctrl Pts',(-43.3012701892219,7.91666666666667,25.));
#20240=CARTESIAN_POINT('Ctrl Pts',(-36.6025403784438,8.125,36.6025403784438));
#20241=CARTESIAN_POINT('Ctrl Pts',(-25.,8.33333333333333,43.3012701892219));
#20242=CARTESIAN_POINT('Ctrl Pts',(-13.3974596215562,8.54166666666667,50.));
#20243=CARTESIAN_POINT('Ctrl Pts',(0.,8.75,50.));
#20244=CARTESIAN_POINT('Ctrl Pts',(13.3974596215562,8.95833333333333,50.));
#20245=CARTESIAN_POINT('Ctrl Pts',(25.,9.16666666666667,43.301270189222));
#20246=CARTESIAN_POINT('Ctrl Pts',(36.6025403784438,9.375,36.6025403784439));
#20247=CARTESIAN_POINT('Ctrl Pts',(43.301270189222,9.58333333333333,25.));
#20248=CARTESIAN_POINT('Ctrl Pts',(50.,9.79166666666667,13.3974596215562));
#20249=CARTESIAN_POINT('Ctrl Pts',(50.,10.,4.33680868994202E-16));
#20250=CARTESIAN_POINT('Ctrl Pts',(50.0000000000001,10.2083333333333,-13.3974596215561));
#20251=CARTESIAN_POINT('Ctrl Pts',(43.301270189222,10.4166666666667,-25.));
#20252=CARTESIAN_POINT('Ctrl Pts',(36.6025403784439,10.625,-36.6025403784439));
#20253=CARTESIAN_POINT('Ctrl Pts',(25.0000000000001,10.8333333333333,-43.3012701892219));
#20254=CARTESIAN_POINT('Ctrl Pts',(13.3974596215562,11.0416666666667,-50.));
#20255=CARTESIAN_POINT('Ctrl Pts',(2.77555756156289E-14,11.25,-50.));
#20256=CARTESIAN_POINT('Ctrl Pts',(-13.3974596215561,11.4583333333333,-50.));
#20257=CARTESIAN_POINT('Ctrl Pts',(-25.,11.6666666666667,-43.301270189222));
#20258=CARTESIAN_POINT('Ctrl Pts',(-36.6025403784439,11.875,-36.6025403784439));
#20259=CARTESIAN_POINT('Ctrl Pts',(-43.3012701892219,12.0833333333333,-25.));
#20260=CARTESIAN_POINT('Ctrl Pts',(-50.,12.2916666666667,-13.3974596215561));
#20261=CARTESIAN_POINT('Ctrl Pts',(-50.,12.5,-5.63785129692462E-15));
#20262=CARTESIAN_POINT('Ctrl Pts',(-50.,12.7083333333333,13.3974596215561));
#20263=CARTESIAN_POINT('Ctrl Pts',(-43.3012701892219,12.9166666666667,25.));
#20264=CARTESIAN_POINT('Ctrl Pts',(-36.6025403784438,13.125,36.6025403784438));
#20265=CARTESIAN_POINT('Ctrl Pts',(-25.,13.3333333333333,43.3012701892219));
#20266=CARTESIAN_POINT('Ctrl Pts',(-13.3974596215562,13.5416666666667,50.));
#20267=CARTESIAN_POINT('Ctrl Pts',(0.,13.75,50.));
#20268=CARTESIAN_POINT('Ctrl Pts',(13.3974596215562,13.9583333333333,50.));
#20269=CARTESIAN_POINT('Ctrl Pts',(25.,14.1666666666667,43.301270189222));
#20270=CARTESIAN_POINT('Ctrl Pts',(36.6025403784438,14.375,36.6025403784439));
#20271=CARTESIAN_POINT('Ctrl Pts',(43.301270189222,14.5833333333333,25.));
#20272=CARTESIAN_POINT('Ctrl Pts',(50.,14.7916666666667,13.3974596215562));
#20273=CARTESIAN_POINT('Ctrl Pts',(50.,15.,4.33680868994202E-16));
#20274=CARTESIAN_POINT('Ctrl Pts',(50.0000000000001,15.2083333333333,-13.3974596215561));
#20275=CARTESIAN_POINT('Ctrl Pts',(43.301270189222,15.4166666666667,-25.));
#20276=CARTESIAN_POINT('Ctrl Pts',(36.6025403784439,15.625,-36.6025403784439));
#20277=CARTESIAN_POINT('Ctrl Pts',(25.0000000000001,15.8333333333333,-43.3012701892219));
#20278=CARTESIAN_POINT('Ctrl Pts',(13.3974596215562,16.0416666666667,-50.));
#20279=CARTESIAN_POINT('Ctrl Pts',(2.77555756156289E-14,16.25,-50.));
#20280=CARTESIAN_POINT('Ctrl Pts',(-13.3974596215561,16.4583333333333,-50.));
#20281=CARTESIAN_POINT('Ctrl Pts',(-25.,16.6666666666667,-43.301270189222));
#20282=CARTESIAN_POINT('Ctrl Pts',(-36.6025403784439,16.875,-36.6025403784439));
#20283=CARTESIAN_POINT('Ctrl Pts',(-43.3012701892219,17.0833333333333,-25.));
#20284=CARTESIAN_POINT('Ctrl Pts',(-50.,17.2916666666667,-13.3974596215561));
#20285=CARTESIAN_POINT('Ctrl Pts',(-50.,17.5,-5.63785129692462E-15));
#20286=CARTESIAN_POINT('Ctrl Pts',(-50.,17.7083333333333,13.3974596215561));
#20287=CARTESIAN_POINT('Ctrl Pts',(-43.3012701892219,17.9166666666667,25.));
#20288=CARTESIAN_POINT('Ctrl Pts',(-36.6025403784438,18.125,36.6025403784438));
#20289=CARTESIAN_POINT('Ctrl Pts',(-25.,18.3333333333333,43.3012701892219));
#20290=CARTESIAN_POINT('Ctrl Pts',(-13.3974596215562,18.5416666666667,50.));
#20291=CARTESIAN_POINT('Ctrl Pts',(0.,18.75,50.));
#20292=CARTESIAN_POINT('Ctrl Pts',(7.91921883571848,18.8731455293798,50.));
#20293=CARTESIAN_POINT('Ctrl Pts',(15.4508438171073,19.0004604433872,47.5528277323164));
#20294=CARTESIAN_POINT('Ctrl Pts',(21.1563918137039,19.0969072731679,45.6989835932745));
#20295=CARTESIAN_POINT('Ctrl Pts',(26.8619398103006,19.1933541029486,43.8451394542326));
#20296=CARTESIAN_POINT('Origin',(0.,26.58,0.));
#20297=CARTESIAN_POINT('Origin',(0.,20.58,0.));
#20298=CARTESIAN_POINT('Origin',(0.,23.58,0.));
#20636=UNCERTAINTY_MEASURE_WITH_UNIT(LENGTH_MEASURE(0.01),#20659,
'DISTANCE_ACCURACY_VALUE',
'Maximum model space distance between geometric entities at asserted c
onnectivities');
#20644=UNCERTAINTY_MEASURE_WITH_UNIT(LENGTH_MEASURE(0.01),#20659,
'DISTANCE_ACCURACY_VALUE',
'Maximum model space distance between geometric entities at asserted c
onnectivities');
#20650=(
GEOMETRIC_REPRESENTATION_CONTEXT(3)
GLOBAL_UNCERTAINTY_ASSIGNED_CONTEXT((#20636))
GLOBAL_UNIT_ASSIGNED_CONTEXT((#20659,#20661,#20662))
REPRESENTATION_CONTEXT('','3D')
);
#20658=(
GEOMETRIC_REPRESENTATION_CONTEXT(3)
GLOBAL_UNCERTAINTY_ASSIGNED_CONTEXT((#20644))
GLOBAL_UNIT_ASSIGNED_CONTEXT((#20659,#20661,#20662))
REPRESENTATION_CONTEXT('','3D')
);
#20659=(
LENGTH_UNIT()
NAMED_UNIT(*)
SI_UNIT(.MILLI.,.METRE.)
);
#20661=(
NAMED_UNIT(*)
PLANE_ANGLE_UNIT()
SI_UNIT($,.RADIAN.)
);
#20662=(
NAMED_UNIT(*)
SI_UNIT($,.STERADIAN.)
SOLID_ANGLE_UNIT()
);
#20668=SHAPE_DEFINITION_REPRESENTATION(#20681,#20720);
#20681=PRODUCT_DEFINITION_SHAPE('',$,#20734);
#20720=SHAPE_REPRESENTATION('',(#3932),#20650);
#20728=PRODUCT_DEFINITION_CONTEXT('part definition',#20769,'design');
#20734=PRODUCT_DEFINITION('cover','Cover',#20747,#20728);
#20747=PRODUCT_DEFINITION_FORMATION('',$,#20776);
#20769=APPLICATION_CONTEXT(
'Core Data for Automotive Mechanical Design Process');
#20770=PRODUCT_CONTEXT('part definition',#20769,'mechanical');
#20776=PRODUCT('cover','Cover',$,(#20770));
#20787=PRESENTATION_STYLE_ASSIGNMENT((#20792));
#20792=SURFACE_STYLE_USAGE(.BOTH.,#20797);
#20797=SURFACE_SIDE_STYLE('',(#20802));
#20802=SURFACE_STYLE_FILL_AREA(#20807);
#20807=FILL_AREA_STYLE('Opaque(227,224,212)',(#20812));
#20812=FILL_AREA_STYLE_COLOUR('Opaque(227,224,212)',#20817);
#20817=COLOUR_RGB('Opaque(227,224,212)',0.890196078431372,0.87843137254902,
0.831372549019608);
ENDSEC;
END-ISO-10303-21;
